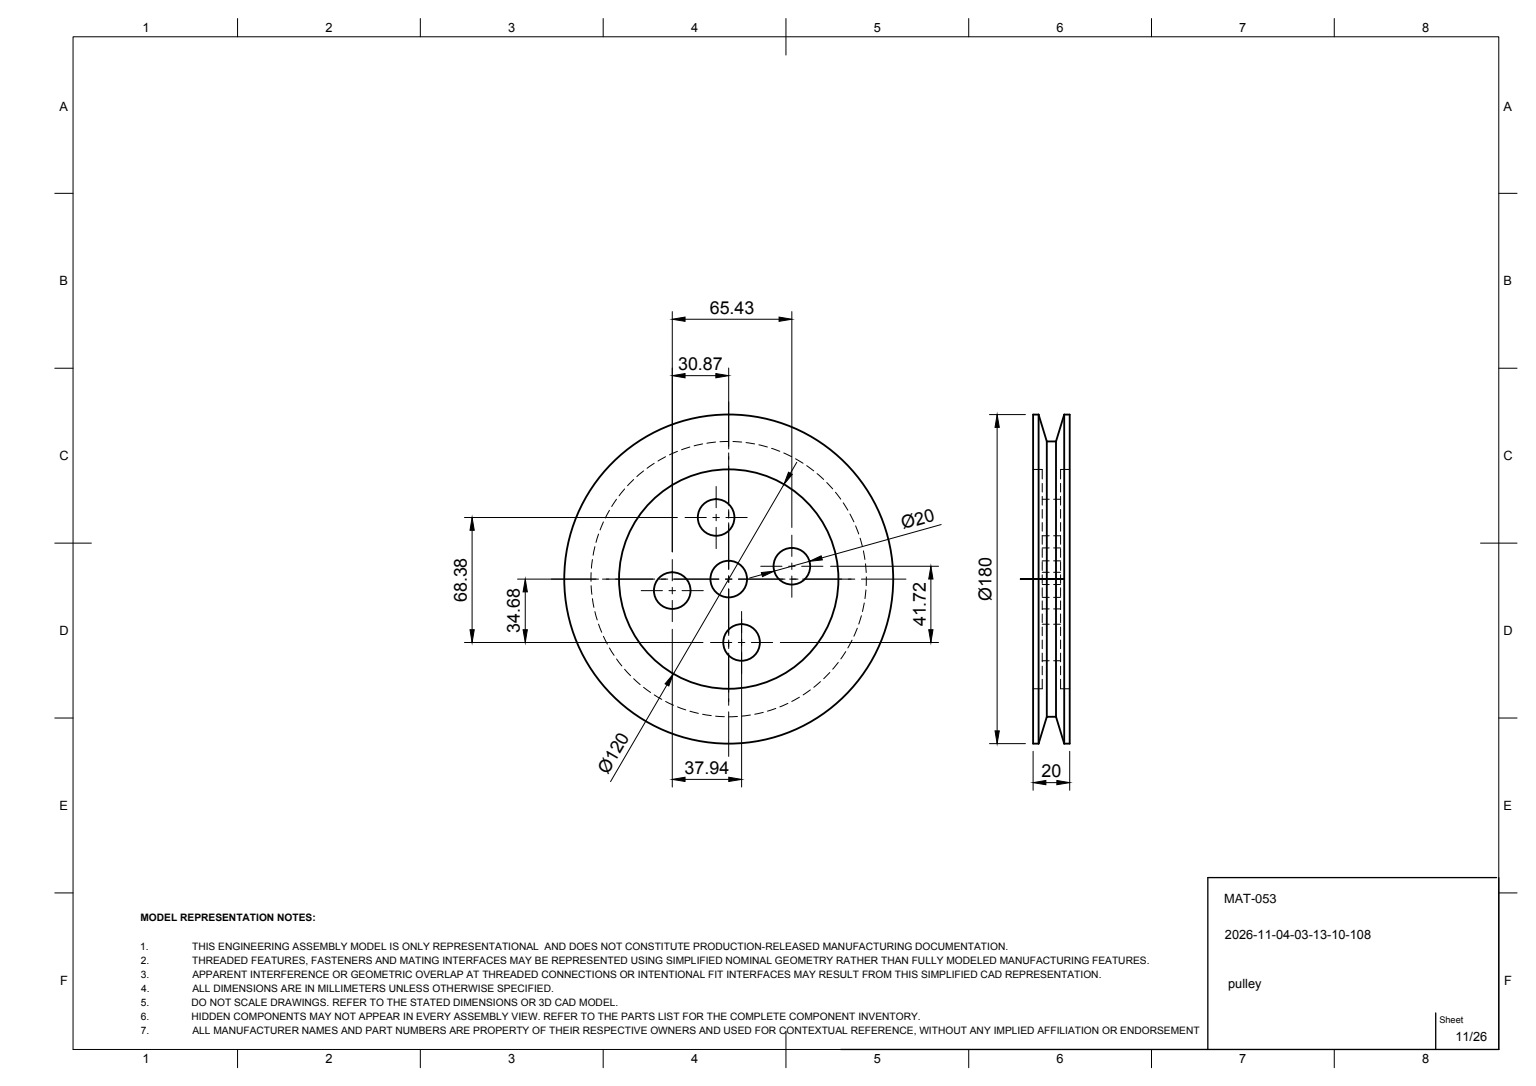
ISO-10303-21;
HEADER;
FILE_DESCRIPTION (('STEP AP214'),
    '1' );
FILE_NAME ('pulley.step',
    '2026-10-10T03:43:58',
    ( '' ),
    ( '' ),
    'SwSTEP 2.0',
    'SolidWorks 2026',
    '' );
FILE_SCHEMA (( 'AUTOMOTIVE_DESIGN' ));
ENDSEC;

DATA;
#61=CYLINDRICAL_SURFACE ( 'NONE', #28597, 10.00000000000000000 ) ;
#98=ORIENTED_EDGE ( 'NONE', *, *, #55652, .T. ) ;
#151=ADVANCED_FACE ( 'NONE', ( #63279 ), #44007, .T. ) ;
#319=CIRCLE ( 'NONE', #56472, 10.00000000000000178 ) ;
#365=AXIS2_PLACEMENT_3D ( 'NONE', #2334, #1994, #61414 ) ;
#474=DIRECTION ( 'NONE',  ( 0.000000000000000000, 0.000000000000000000, 1.000000000000000000 ) ) ;
#651=DIRECTION ( 'NONE',  ( -1.000000000000000000, 0.000000000000000000, 0.000000000000000000 ) ) ;
#941=EDGE_CURVE ( 'NONE', #52293, #21319, #16043, .T. ) ;
#1200=ORIENTED_EDGE ( 'NONE', *, *, #38790, .T. ) ;
#1261=DIRECTION ( 'NONE',  ( 0.000000000000000000, 0.000000000000000000, 1.000000000000000000 ) ) ;
#1262=EDGE_CURVE ( 'NONE', #23524, #39998, #319, .T. ) ;
#1394=( NAMED_UNIT ( * ) SI_UNIT ( $, .STERADIAN. ) SOLID_ANGLE_UNIT ( ) );
#1416=CARTESIAN_POINT ( 'NONE',  ( 0.000000000000000000, 35.26862320190615208, -9.999999999999998224 ) ) ;
#1462=CARTESIAN_POINT ( 'NONE',  ( 89.99999999999998579, 0.000000000000000000, 7.000000000000000000 ) ) ;
#1503=EDGE_LOOP ( 'NONE', ( #64737, #47138, #56812, #9323 ) ) ;
#1529=LINE ( 'NONE', #55690, #24184 ) ;
#1565=MECHANICAL_DESIGN_GEOMETRIC_PRESENTATION_REPRESENTATION('',(#34171),#59945);
#1694=EDGE_CURVE ( 'NONE', #53100, #28536, #21713, .T. ) ;
#1730=AXIS2_PLACEMENT_3D ( 'NONE', #16357, #31849, #58564 ) ;
#1752=FILL_AREA_STYLE ('',( #65780 ) ) ;
#1861=CARTESIAN_POINT ( 'NONE',  ( 0.000000000000000000, 0.000000000000000000, 10.00000000000000000 ) ) ;
#1994=DIRECTION ( 'NONE',  ( -0.000000000000000000, -0.000000000000000000, 1.000000000000000000 ) ) ;
#2049=DIRECTION ( 'NONE',  ( 1.000000000000000000, 0.000000000000000000, 0.000000000000000000 ) ) ;
#2163=EDGE_CURVE ( 'NONE', #30662, #53211, #9601, .T. ) ;
#2167=DIRECTION ( 'NONE',  ( 0.000000000000000000, 0.000000000000000000, 1.000000000000000000 ) ) ;
#2236=EDGE_CURVE ( 'NONE', #53211, #61781, #59915, .T. ) ;
#2298=AXIS2_PLACEMENT_3D ( 'NONE', #8382, #19975, #61496 ) ;
#2334=CARTESIAN_POINT ( 'NONE',  ( 0.000000000000000000, 0.000000000000000000, 2.500000000000030198 ) ) ;
#2371=EDGE_LOOP ( 'NONE', ( #59908, #20323, #39063, #20263 ) ) ;
#2403=VERTEX_POINT ( 'NONE', #29243 ) ;
#2428=CARTESIAN_POINT ( 'NONE',  ( -60.00000000000000000, 0.000000000000000000, -10.00000000000000000 ) ) ;
#2431=EDGE_LOOP ( 'NONE', ( #44600, #48576 ) ) ;
#2555=DIRECTION ( 'NONE',  ( 1.000000000000000000, 0.000000000000000000, 0.000000000000000000 ) ) ;
#2581=ORIENTED_EDGE ( 'NONE', *, *, #47265, .T. ) ;
#2644=ORIENTED_EDGE ( 'NONE', *, *, #1262, .F. ) ;
#2646=CIRCLE ( 'NONE', #56567, 60.00000000000000000 ) ;
#2656=DIRECTION ( 'NONE',  ( 0.000000000000000000, 0.000000000000000000, 1.000000000000000000 ) ) ;
#2718=DIRECTION ( 'NONE',  ( 1.000000000000000000, 0.000000000000000000, 0.000000000000000000 ) ) ;
#2740=AXIS2_PLACEMENT_3D ( 'NONE', #51849, #29706, #19145 ) ;
#2780=EDGE_CURVE ( 'NONE', #47684, #28536, #39364, .T. ) ;
#2790=ORIENTED_EDGE ( 'NONE', *, *, #64406, .T. ) ;
#2793=AXIS2_PLACEMENT_3D ( 'NONE', #21535, #48592, #64454 ) ;
#2893=VERTEX_POINT ( 'NONE', #68763 ) ;
#3121=EDGE_CURVE ( 'NONE', #10742, #65175, #4948, .T. ) ;
#3254=ADVANCED_FACE ( 'NONE', ( #52841, #58140 ), #58814, .F. ) ;
#3361=CARTESIAN_POINT ( 'NONE',  ( -10.00000000000000178, -31.50328976398030534, -5.000000000000000000 ) ) ;
#3370=ORIENTED_EDGE ( 'NONE', *, *, #2236, .F. ) ;
#3553=ORIENTED_EDGE ( 'NONE', *, *, #22471, .F. ) ;
#3589=VECTOR ( 'NONE', #31637, 1000.000000000000000 ) ;
#3744=EDGE_LOOP ( 'NONE', ( #59233, #13673, #7017, #48460 ) ) ;
#3816=CARTESIAN_POINT ( 'NONE',  ( 0.000000000000000000, 0.000000000000000000, -5.000000000000000000 ) ) ;
#3870=ORIENTED_EDGE ( 'NONE', *, *, #47160, .T. ) ;
#4067=DIRECTION ( 'NONE',  ( -0.000000000000000000, -0.000000000000000000, 1.000000000000000000 ) ) ;
#4088=SHAPE_DEFINITION_REPRESENTATION ( #20886, #7414 ) ;
#4166=FACE_BOUND ( 'NONE', #26669, .T. ) ;
#4396=CARTESIAN_POINT ( 'NONE',  ( 0.000000000000000000, 35.26862320190615208, -5.000000000000000000 ) ) ;
#4448=DIRECTION ( 'NONE',  ( -0.000000000000000000, -0.000000000000000000, -1.000000000000000000 ) ) ;
#4451=ORIENTED_EDGE ( 'NONE', *, *, #11819, .F. ) ;
#4637=AXIS2_PLACEMENT_3D ( 'NONE', #21081, #17074, #49079 ) ;
#4684=AXIS2_PLACEMENT_3D ( 'NONE', #58250, #22002, #20968 ) ;
#4704=EDGE_CURVE ( 'NONE', #10742, #21319, #42324, .T. ) ;
#4769=EDGE_LOOP ( 'NONE', ( #6850, #46312, #5479, #66133 ) ) ;
#4782=CARTESIAN_POINT ( 'NONE',  ( 0.000000000000000000, 0.000000000000000000, 2.500000000000030198 ) ) ;
#4843=FACE_OUTER_BOUND ( 'NONE', #65401, .T. ) ;
#4888=VECTOR ( 'NONE', #64816, 1000.000000000000000 ) ;
#4897=EDGE_CURVE ( 'NONE', #66948, #13402, #48184, .T. ) ;
#4914=EDGE_CURVE ( 'NONE', #2403, #18591, #2646, .T. ) ;
#4948=CIRCLE ( 'NONE', #10407, 10.00000000000000178 ) ;
#5011=CARTESIAN_POINT ( 'NONE',  ( 0.000000000000000000, 0.000000000000000000, -10.00000000000000000 ) ) ;
#5069=ORIENTED_EDGE ( 'NONE', *, *, #52323, .T. ) ;
#5081=CARTESIAN_POINT ( 'NONE',  ( 35.39413431650373099, 0.000000000000000000, -9.999999999999998224 ) ) ;
#5354=DIRECTION ( 'NONE',  ( 1.000000000000000000, 0.000000000000000000, 0.000000000000000000 ) ) ;
#5479=ORIENTED_EDGE ( 'NONE', *, *, #19013, .F. ) ;
#5630=CARTESIAN_POINT ( 'NONE',  ( 89.99999999999998579, 0.000000000000000000, 7.000000000000000000 ) ) ;
#5730=AXIS2_PLACEMENT_3D ( 'NONE', #1861, #22599, #60236 ) ;
#5982=VECTOR ( 'NONE', #10217, 999.9999999999998863 ) ;
#6135=AXIS2_PLACEMENT_3D ( 'NONE', #10751, #4448, #36807 ) ;
#6243=ORIENTED_EDGE ( 'NONE', *, *, #19527, .T. ) ;
#6270=ORIENTED_EDGE ( 'NONE', *, *, #4897, .F. ) ;
#6271=EDGE_LOOP ( 'NONE', ( #58574, #4451 ) ) ;
#6334=DIRECTION ( 'NONE',  ( 0.000000000000000000, 0.000000000000000000, 1.000000000000000000 ) ) ;
#6410=ADVANCED_FACE ( 'NONE', ( #50308 ), #22872, .F. ) ;
#6426=ORIENTED_EDGE ( 'NONE', *, *, #48732, .T. ) ;
#6486=AXIS2_PLACEMENT_3D ( 'NONE', #11579, #27769, #7377 ) ;
#6559=LINE ( 'NONE', #26464, #41857 ) ;
#6569=DIRECTION ( 'NONE',  ( 1.000000000000000000, 0.000000000000000000, 0.000000000000000000 ) ) ;
#6575=CYLINDRICAL_SURFACE ( 'NONE', #36283, 10.00000000000000178 ) ;
#6794=VERTEX_POINT ( 'NONE', #69156 ) ;
#6834=CARTESIAN_POINT ( 'NONE',  ( 0.000000000000000000, -31.50328976398030534, -9.999999999999998224 ) ) ;
#6850=ORIENTED_EDGE ( 'NONE', *, *, #7053, .T. ) ;
#6887=CARTESIAN_POINT ( 'NONE',  ( 89.99999999999998579, 0.000000000000000000, -7.000000000000000000 ) ) ;
#6996=LINE ( 'NONE', #34089, #60070 ) ;
#7017=ORIENTED_EDGE ( 'NONE', *, *, #941, .T. ) ;
#7039=DIRECTION ( 'NONE',  ( -0.000000000000000000, -0.000000000000000000, 1.000000000000000000 ) ) ;
#7047=EDGE_CURVE ( 'NONE', #45363, #9869, #62339, .T. ) ;
#7053=EDGE_CURVE ( 'NONE', #68618, #30662, #37622, .T. ) ;
#7236=EDGE_CURVE ( 'NONE', #21145, #17425, #50034, .T. ) ;
#7241=DIRECTION ( 'NONE',  ( 1.000000000000000000, 0.000000000000000000, 0.000000000000000000 ) ) ;
#7247=ORIENTED_EDGE ( 'NONE', *, *, #41042, .T. ) ;
#7317=AXIS2_PLACEMENT_3D ( 'NONE', #58860, #10002, #69423 ) ;
#7333=ORIENTED_EDGE ( 'NONE', *, *, #46538, .F. ) ;
#7377=DIRECTION ( 'NONE',  ( 1.000000000000000000, 0.000000000000000000, 0.000000000000000000 ) ) ;
#7414=SHAPE_REPRESENTATION ( 'pulley', ( #66832 ), #23071 ) ;
#7453=DIRECTION ( 'NONE',  ( 1.000000000000000000, 0.000000000000000000, 0.000000000000000000 ) ) ;
#7463=EDGE_CURVE ( 'NONE', #12451, #43150, #55952, .T. ) ;
#7697=AXIS2_PLACEMENT_3D ( 'NONE', #38245, #42146, #53030 ) ;
#7758=DIRECTION ( 'NONE',  ( 1.000000000000000000, 0.000000000000000000, 0.000000000000000000 ) ) ;
#7775=CARTESIAN_POINT ( 'NONE',  ( -44.39004539972346208, 1.224646799147353059E-15, 5.000000000000000000 ) ) ;
#7976=EDGE_LOOP ( 'NONE', ( #6270, #47375, #12404, #6426 ) ) ;
#8319=DIRECTION ( 'NONE',  ( 1.000000000000000000, 0.000000000000000000, 0.000000000000000000 ) ) ;
#8359=ADVANCED_FACE ( 'NONE', ( #59050, #26025, #42538, #37948, #37249, #31988 ), #26369, .T. ) ;
#8382=CARTESIAN_POINT ( 'NONE',  ( 0.000000000000000000, 0.000000000000000000, -50.00000000000000711 ) ) ;
#8432=ADVANCED_FACE ( 'NONE', ( #11546 ), #33731, .F. ) ;
#8454=CARTESIAN_POINT ( 'NONE',  ( -34.39004539972345498, 0.000000000000000000, -9.999999999999998224 ) ) ;
#8513=CARTESIAN_POINT ( 'NONE',  ( 89.99999999999998579, 0.000000000000000000, 10.00000000000000000 ) ) ;
#8624=EDGE_CURVE ( 'NONE', #11248, #10057, #61672, .T. ) ;
#8655=ORIENTED_EDGE ( 'NONE', *, *, #46300, .T. ) ;
#8682=ORIENTED_EDGE ( 'NONE', *, *, #41042, .F. ) ;
#8921=AXIS2_PLACEMENT_3D ( 'NONE', #60437, #34420, #651 ) ;
#8935=ORIENTED_EDGE ( 'NONE', *, *, #27892, .T. ) ;
#9037=CARTESIAN_POINT ( 'NONE',  ( 0.000000000000000000, -31.50328976398030534, 5.000000000000000000 ) ) ;
#9296=DIRECTION ( 'NONE',  ( -0.000000000000000000, -0.000000000000000000, 1.000000000000000000 ) ) ;
#9299=CARTESIAN_POINT ( 'NONE',  ( -60.00000000000000000, 7.347880794884118356E-15, 5.000000000000000000 ) ) ;
#9323=ORIENTED_EDGE ( 'NONE', *, *, #67194, .F. ) ;
#9353=ADVANCED_FACE ( 'NONE', ( #51360 ), #35525, .T. ) ;
#9510=DIRECTION ( 'NONE',  ( 0.000000000000000000, 0.000000000000000000, 1.000000000000000000 ) ) ;
#9547=VERTEX_POINT ( 'NONE', #49508 ) ;
#9601=LINE ( 'NONE', #31064, #27333 ) ;
#9685=ORIENTED_EDGE ( 'NONE', *, *, #17023, .T. ) ;
#9689=DIRECTION ( 'NONE',  ( 0.000000000000000000, 0.000000000000000000, 1.000000000000000000 ) ) ;
#9869=VERTEX_POINT ( 'NONE', #16396 ) ;
#10002=DIRECTION ( 'NONE',  ( -0.000000000000000000, -0.000000000000000000, 1.000000000000000000 ) ) ;
#10051=VECTOR ( 'NONE', #40595, 1000.000000000000000 ) ;
#10057=VERTEX_POINT ( 'NONE', #36395 ) ;
#10178=CARTESIAN_POINT ( 'NONE',  ( 0.000000000000000000, 0.000000000000000000, 5.000000000000000000 ) ) ;
#10217=DIRECTION ( 'NONE',  ( 0.9561276726666709802, 1.170918693907447064E-16, -0.2929502919626733037 ) ) ;
#10257=AXIS2_PLACEMENT_3D ( 'NONE', #8454, #17612, #17965 ) ;
#10407=AXIS2_PLACEMENT_3D ( 'NONE', #35304, #56760, #35656 ) ;
#10513=DIRECTION ( 'NONE',  ( 1.000000000000000000, 0.000000000000000000, 0.000000000000000000 ) ) ;
#10545=ORIENTED_EDGE ( 'NONE', *, *, #941, .F. ) ;
#10712=LINE ( 'NONE', #53950, #37950 ) ;
#10742=VERTEX_POINT ( 'NONE', #35449 ) ;
#10751=CARTESIAN_POINT ( 'NONE',  ( 0.000000000000000000, 0.000000000000000000, -5.000000000000000000 ) ) ;
#10829=EDGE_LOOP ( 'NONE', ( #67970, #52613, #98, #33206 ) ) ;
#10892=ORIENTED_EDGE ( 'NONE', *, *, #33419, .T. ) ;
#11059=CARTESIAN_POINT ( 'NONE',  ( -10.00000000000000000, 1.224646799147353256E-15, -50.00000000000000711 ) ) ;
#11248=VERTEX_POINT ( 'NONE', #3361 ) ;
#11305=CARTESIAN_POINT ( 'NONE',  ( 0.000000000000000000, 0.000000000000000000, -50.00000000000000711 ) ) ;
#11354=DIRECTION ( 'NONE',  ( 1.000000000000000000, 0.000000000000000000, 0.000000000000000000 ) ) ;
#11546=FACE_OUTER_BOUND ( 'NONE', #63868, .T. ) ;
#11579=CARTESIAN_POINT ( 'NONE',  ( 0.000000000000000000, 0.000000000000000000, -10.00000000000000000 ) ) ;
#11681=ORIENTED_EDGE ( 'NONE', *, *, #47864, .F. ) ;
#11757=DIRECTION ( 'NONE',  ( 1.000000000000000000, 0.000000000000000000, 0.000000000000000000 ) ) ;
#11819=EDGE_CURVE ( 'NONE', #30259, #53637, #18799, .T. ) ;
#11950=DIRECTION ( 'NONE',  ( -0.000000000000000000, -0.000000000000000000, 1.000000000000000000 ) ) ;
#12100=EDGE_CURVE ( 'NONE', #2893, #44947, #27719, .T. ) ;
#12102=DIRECTION ( 'NONE',  ( 1.000000000000000000, 0.000000000000000000, 0.000000000000000000 ) ) ;
#12106=ORIENTED_EDGE ( 'NONE', *, *, #38790, .F. ) ;
#12276=CARTESIAN_POINT ( 'NONE',  ( 0.000000000000000000, 0.000000000000000000, -5.000000000000000000 ) ) ;
#12300=SURFACE_STYLE_FILL_AREA ( #1752 ) ;
#12372=FACE_OUTER_BOUND ( 'NONE', #13779, .T. ) ;
#12404=ORIENTED_EDGE ( 'NONE', *, *, #67194, .T. ) ;
#12410=ORIENTED_EDGE ( 'NONE', *, *, #55652, .F. ) ;
#12451=VERTEX_POINT ( 'NONE', #50090 ) ;
#12519=CARTESIAN_POINT ( 'NONE',  ( -34.39004539972345498, 0.000000000000000000, 5.000000000000000000 ) ) ;
#12551=FACE_OUTER_BOUND ( 'NONE', #3744, .T. ) ;
#12617=EDGE_LOOP ( 'NONE', ( #21075, #40042 ) ) ;
#12653=PRESENTATION_STYLE_ASSIGNMENT (( #29179 ) ) ;
#12808=EDGE_LOOP ( 'NONE', ( #2644, #35837 ) ) ;
#12934=CARTESIAN_POINT ( 'NONE',  ( 0.000000000000000000, -31.50328976398030534, -9.999999999999998224 ) ) ;
#13038=CIRCLE ( 'NONE', #25394, 10.00000000000000178 ) ;
#13049=FACE_OUTER_BOUND ( 'NONE', #2371, .T. ) ;
#13176=CIRCLE ( 'NONE', #36765, 60.00000000000000000 ) ;
#13196=ORIENTED_EDGE ( 'NONE', *, *, #60306, .F. ) ;
#13220=DIRECTION ( 'NONE',  ( 1.000000000000000000, 0.000000000000000000, 0.000000000000000000 ) ) ;
#13374=CARTESIAN_POINT ( 'NONE',  ( -89.99999999999998579, 1.102182119232617596E-14, 7.000000000000000000 ) ) ;
#13402=VERTEX_POINT ( 'NONE', #6887 ) ;
#13464=VECTOR ( 'NONE', #31449, 1000.000000000000000 ) ;
#13673=ORIENTED_EDGE ( 'NONE', *, *, #49690, .T. ) ;
#13697=LINE ( 'NONE', #49932, #55890 ) ;
#13724=CARTESIAN_POINT ( 'NONE',  ( 10.00000000000000178, -31.50328976398030534, -9.999999999999998224 ) ) ;
#13779=EDGE_LOOP ( 'NONE', ( #39660, #49194, #20199, #56429 ) ) ;
#13918=EDGE_LOOP ( 'NONE', ( #29003, #10892, #68043, #19610 ) ) ;
#13923=CARTESIAN_POINT ( 'NONE',  ( -75.31295361348102801, 9.223176757708264319E-15, 2.500000000000030198 ) ) ;
#14038=VECTOR ( 'NONE', #9296, 1000.000000000000000 ) ;
#14075=EDGE_CURVE ( 'NONE', #50425, #20755, #16062, .T. ) ;
#14430=AXIS2_PLACEMENT_3D ( 'NONE', #16488, #59392, #10513 ) ;
#14504=ADVANCED_FACE ( 'NONE', ( #20920 ), #64168, .F. ) ;
#14523=CIRCLE ( 'NONE', #25733, 10.00000000000000178 ) ;
#14612=DIRECTION ( 'NONE',  ( 1.000000000000000000, 0.000000000000000000, 0.000000000000000000 ) ) ;
#14735=DIRECTION ( 'NONE',  ( -0.000000000000000000, -0.000000000000000000, 1.000000000000000000 ) ) ;
#14817=AXIS2_PLACEMENT_3D ( 'NONE', #9037, #51934, #2718 ) ;
#14996=CYLINDRICAL_SURFACE ( 'NONE', #6135, 60.00000000000000000 ) ;
#15212=LINE ( 'NONE', #52828, #51280 ) ;
#15564=DIRECTION ( 'NONE',  ( -0.000000000000000000, -0.000000000000000000, 1.000000000000000000 ) ) ;
#15578=PRODUCT_DEFINITION_CONTEXT ( 'detailed design', #55716, 'design' ) ;
#15691=FACE_OUTER_BOUND ( 'NONE', #46295, .T. ) ;
#15971=DIRECTION ( 'NONE',  ( -1.000000000000000000, 0.000000000000000000, 0.000000000000000000 ) ) ;
#16043=CIRCLE ( 'NONE', #57638, 10.00000000000000178 ) ;
#16062=LINE ( 'NONE', #58619, #49377 ) ;
#16244=EDGE_CURVE ( 'NONE', #6794, #27439, #31571, .T. ) ;
#16357=CARTESIAN_POINT ( 'NONE',  ( 0.000000000000000000, 0.000000000000000000, -10.00000000000000000 ) ) ;
#16396=CARTESIAN_POINT ( 'NONE',  ( -89.99999999999998579, 1.102182119232617596E-14, -10.00000000000000000 ) ) ;
#16488=CARTESIAN_POINT ( 'NONE',  ( 0.000000000000000000, 0.000000000000000000, -10.00000000000000000 ) ) ;
#16557=AXIS2_PLACEMENT_3D ( 'NONE', #18172, #45239, #6569 ) ;
#16580=ORIENTED_EDGE ( 'NONE', *, *, #2780, .F. ) ;
#16619=AXIS2_PLACEMENT_3D ( 'NONE', #39594, #2656, #40976 ) ;
#16620=ORIENTED_EDGE ( 'NONE', *, *, #51700, .F. ) ;
#16686=EDGE_CURVE ( 'NONE', #66948, #47684, #54082, .T. ) ;
#16809=LINE ( 'NONE', #49156, #47554 ) ;
#17023=EDGE_CURVE ( 'NONE', #44947, #9547, #6996, .T. ) ;
#17037=CYLINDRICAL_SURFACE ( 'NONE', #1730, 89.99999999999998579 ) ;
#17074=DIRECTION ( 'NONE',  ( 0.000000000000000000, 0.000000000000000000, 1.000000000000000000 ) ) ;
#17125=AXIS2_PLACEMENT_3D ( 'NONE', #54806, #50934, #23164 ) ;
#17213=CARTESIAN_POINT ( 'NONE',  ( 60.00000000000000000, 0.000000000000000000, 5.000000000000000000 ) ) ;
#17290=CARTESIAN_POINT ( 'NONE',  ( 35.39413431650373099, 0.000000000000000000, -5.000000000000000000 ) ) ;
#17382=FACE_OUTER_BOUND ( 'NONE', #10829, .T. ) ;
#17425=VERTEX_POINT ( 'NONE', #61678 ) ;
#17612=DIRECTION ( 'NONE',  ( -0.000000000000000000, -0.000000000000000000, 1.000000000000000000 ) ) ;
#17645=DIRECTION ( 'NONE',  ( 1.000000000000000000, 0.000000000000000000, 0.000000000000000000 ) ) ;
#17965=DIRECTION ( 'NONE',  ( 1.000000000000000000, 0.000000000000000000, 0.000000000000000000 ) ) ;
#18029=DIRECTION ( 'NONE',  ( 0.000000000000000000, 0.000000000000000000, 1.000000000000000000 ) ) ;
#18172=CARTESIAN_POINT ( 'NONE',  ( 0.000000000000000000, 0.000000000000000000, -10.00000000000000000 ) ) ;
#18202=EDGE_CURVE ( 'NONE', #17425, #2403, #29517, .T. ) ;
#18545=ORIENTED_EDGE ( 'NONE', *, *, #34312, .F. ) ;
#18587=CONICAL_SURFACE ( 'NONE', #42136, 75.31295361348104223, 1.273485274044411586 ) ;
#18591=VERTEX_POINT ( 'NONE', #67778 ) ;
#18605=ORIENTED_EDGE ( 'NONE', *, *, #3121, .F. ) ;
#18616=VECTOR ( 'NONE', #52054, 1000.000000000000000 ) ;
#18687=CARTESIAN_POINT ( 'NONE',  ( 0.000000000000000000, 0.000000000000000000, 10.00000000000000000 ) ) ;
#18709=VECTOR ( 'NONE', #66024, 1000.000000000000000 ) ;
#18799=CIRCLE ( 'NONE', #42345, 10.00000000000000178 ) ;
#18919=CARTESIAN_POINT ( 'NONE',  ( 10.00000000000000178, -31.50328976398030534, 5.000000000000000000 ) ) ;
#18926=CARTESIAN_POINT ( 'NONE',  ( -60.00000000000000000, 7.347880794884118356E-15, 5.000000000000000000 ) ) ;
#18993=CARTESIAN_POINT ( 'NONE',  ( 0.000000000000000000, 0.000000000000000000, 10.00000000000000000 ) ) ;
#19013=EDGE_CURVE ( 'NONE', #61781, #53211, #19248, .T. ) ;
#19145=DIRECTION ( 'NONE',  ( 1.000000000000000000, 0.000000000000000000, 0.000000000000000000 ) ) ;
#19248=CIRCLE ( 'NONE', #5730, 89.99999999999998579 ) ;
#19463=EDGE_CURVE ( 'NONE', #20755, #30529, #57469, .T. ) ;
#19525=DIRECTION ( 'NONE',  ( 0.000000000000000000, 0.000000000000000000, 1.000000000000000000 ) ) ;
#19527=EDGE_CURVE ( 'NONE', #47684, #66948, #67617, .T. ) ;
#19586=EDGE_CURVE ( 'NONE', #28536, #53100, #60827, .T. ) ;
#19610=ORIENTED_EDGE ( 'NONE', *, *, #18202, .F. ) ;
#19678=DIRECTION ( 'NONE',  ( 0.000000000000000000, 0.000000000000000000, 1.000000000000000000 ) ) ;
#19778=DIRECTION ( 'NONE',  ( 0.000000000000000000, 0.000000000000000000, 1.000000000000000000 ) ) ;
#19800=CIRCLE ( 'NONE', #46751, 60.00000000000000000 ) ;
#19975=DIRECTION ( 'NONE',  ( -0.000000000000000000, -0.000000000000000000, 1.000000000000000000 ) ) ;
#20066=CARTESIAN_POINT ( 'NONE',  ( 35.39413431650373099, 0.000000000000000000, 5.000000000000000000 ) ) ;
#20199=ORIENTED_EDGE ( 'NONE', *, *, #18202, .T. ) ;
#20233=DIRECTION ( 'NONE',  ( -1.000000000000000000, 0.000000000000000000, 0.000000000000000000 ) ) ;
#20263=ORIENTED_EDGE ( 'NONE', *, *, #40347, .T. ) ;
#20321=AXIS2_PLACEMENT_3D ( 'NONE', #4396, #36753, #36062 ) ;
#20323=ORIENTED_EDGE ( 'NONE', *, *, #34312, .T. ) ;
#20358=EDGE_LOOP ( 'NONE', ( #40227, #3870 ) ) ;
#20755=VERTEX_POINT ( 'NONE', #40805 ) ;
#20828=ORIENTED_EDGE ( 'NONE', *, *, #47858, .T. ) ;
#20886=PRODUCT_DEFINITION_SHAPE ( 'NONE', 'NONE',  #57716 ) ;
#20920=FACE_OUTER_BOUND ( 'NONE', #24665, .T. ) ;
#20955=EDGE_CURVE ( 'NONE', #39170, #22725, #44086, .T. ) ;
#20968=DIRECTION ( 'NONE',  ( 1.000000000000000000, 0.000000000000000000, 0.000000000000000000 ) ) ;
#21075=ORIENTED_EDGE ( 'NONE', *, *, #7047, .F. ) ;
#21081=CARTESIAN_POINT ( 'NONE',  ( 0.000000000000000000, 0.000000000000000000, 5.000000000000000000 ) ) ;
#21136=ORIENTED_EDGE ( 'NONE', *, *, #19463, .F. ) ;
#21145=VERTEX_POINT ( 'NONE', #18926 ) ;
#21198=DIRECTION ( 'NONE',  ( 1.000000000000000000, 0.000000000000000000, -0.000000000000000000 ) ) ;
#21199=CIRCLE ( 'NONE', #60511, 10.00000000000000000 ) ;
#21283=DIRECTION ( 'NONE',  ( -1.000000000000000000, 0.000000000000000000, 0.000000000000000000 ) ) ;
#21319=VERTEX_POINT ( 'NONE', #63564 ) ;
#21446=AXIS2_PLACEMENT_3D ( 'NONE', #60287, #64868, #12102 ) ;
#21521=DIRECTION ( 'NONE',  ( 0.000000000000000000, 0.000000000000000000, 1.000000000000000000 ) ) ;
#21535=CARTESIAN_POINT ( 'NONE',  ( 0.000000000000000000, 0.000000000000000000, 7.000000000000000000 ) ) ;
#21581=CARTESIAN_POINT ( 'NONE',  ( 60.00000000000000000, 7.347880794884118356E-15, -5.000000000000000000 ) ) ;
#21713=CIRCLE ( 'NONE', #365, 75.31295361348102801 ) ;
#21837=ADVANCED_FACE ( 'NONE', ( #24401 ), #47815, .F. ) ;
#21846=CYLINDRICAL_SURFACE ( 'NONE', #31458, 89.99999999999998579 ) ;
#21868=EDGE_LOOP ( 'NONE', ( #34452, #7247, #37847, #29975 ) ) ;
#22002=DIRECTION ( 'NONE',  ( -0.000000000000000000, -0.000000000000000000, 1.000000000000000000 ) ) ;
#22054=DIRECTION ( 'NONE',  ( 1.000000000000000000, 0.000000000000000000, 0.000000000000000000 ) ) ;
#22124=CARTESIAN_POINT ( 'NONE',  ( 0.000000000000000000, 0.000000000000000000, -5.000000000000000000 ) ) ;
#22395=VECTOR ( 'NONE', #29536, 1000.000000000000227 ) ;
#22413=CIRCLE ( 'NONE', #8921, 10.00000000000000178 ) ;
#22471=EDGE_CURVE ( 'NONE', #30662, #68618, #37511, .T. ) ;
#22485=ORIENTED_EDGE ( 'NONE', *, *, #41632, .F. ) ;
#22599=DIRECTION ( 'NONE',  ( 0.000000000000000000, 0.000000000000000000, 1.000000000000000000 ) ) ;
#22637=FACE_OUTER_BOUND ( 'NONE', #1503, .T. ) ;
#22725=VERTEX_POINT ( 'NONE', #58137 ) ;
#22787=EDGE_LOOP ( 'NONE', ( #28842, #20828, #57321, #33604 ) ) ;
#22810=DIRECTION ( 'NONE',  ( -1.000000000000000000, 0.000000000000000000, 0.000000000000000000 ) ) ;
#22872=CYLINDRICAL_SURFACE ( 'NONE', #58908, 10.00000000000000178 ) ;
#22964=AXIS2_PLACEMENT_3D ( 'NONE', #60027, #66039, #32956 ) ;
#23071=( GEOMETRIC_REPRESENTATION_CONTEXT ( 3 ) GLOBAL_UNCERTAINTY_ASSIGNED_CONTEXT ( ( #68356 ) ) GLOBAL_UNIT_ASSIGNED_CONTEXT ( ( #36345, #41619, #46543 ) ) REPRESENTATION_CONTEXT ( 'NONE', 'WORKASPACE' ) );
#23164=DIRECTION ( 'NONE',  ( -1.000000000000000000, 0.000000000000000000, 0.000000000000000000 ) ) ;
#23251=CYLINDRICAL_SURFACE ( 'NONE', #10257, 10.00000000000000178 ) ;
#23524=VERTEX_POINT ( 'NONE', #38498 ) ;
#23619=DIRECTION ( 'NONE',  ( 1.000000000000000000, 0.000000000000000000, 0.000000000000000000 ) ) ;
#23675=ORIENTED_EDGE ( 'NONE', *, *, #64054, .F. ) ;
#23979=DIRECTION ( 'NONE',  ( 0.000000000000000000, 0.000000000000000000, -1.000000000000000000 ) ) ;
#24000=LINE ( 'NONE', #60933, #30651 ) ;
#24087=ORIENTED_EDGE ( 'NONE', *, *, #64141, .T. ) ;
#24106=LINE ( 'NONE', #57489, #14038 ) ;
#24184=VECTOR ( 'NONE', #55334, 1000.000000000000000 ) ;
#24314=ADVANCED_FACE ( 'NONE', ( #58147 ), #44339, .T. ) ;
#24401=FACE_OUTER_BOUND ( 'NONE', #39768, .T. ) ;
#24665=EDGE_LOOP ( 'NONE', ( #43122, #49749, #68545, #49224 ) ) ;
#24720=DIRECTION ( 'NONE',  ( 1.000000000000000000, 0.000000000000000000, 0.000000000000000000 ) ) ;
#24744=DIRECTION ( 'NONE',  ( -1.000000000000000000, 0.000000000000000000, 0.000000000000000000 ) ) ;
#24810=CARTESIAN_POINT ( 'NONE',  ( 0.000000000000000000, 0.000000000000000000, -7.000000000000000000 ) ) ;
#24873=CARTESIAN_POINT ( 'NONE',  ( -10.00000000000000000, 1.224646799147353256E-15, -4.999999999999997335 ) ) ;
#24889=ADVANCED_FACE ( 'NONE', ( #64197 ), #17037, .T. ) ;
#25312=ORIENTED_EDGE ( 'NONE', *, *, #16244, .T. ) ;
#25394=AXIS2_PLACEMENT_3D ( 'NONE', #26904, #42732, #21283 ) ;
#25533=DIRECTION ( 'NONE',  ( 1.000000000000000000, 0.000000000000000000, 0.000000000000000000 ) ) ;
#25733=AXIS2_PLACEMENT_3D ( 'NONE', #66482, #65782, #29181 ) ;
#25747=EDGE_CURVE ( 'NONE', #53100, #68618, #59439, .T. ) ;
#25871=CARTESIAN_POINT ( 'NONE',  ( 0.000000000000000000, 0.000000000000000000, 7.000000000000000000 ) ) ;
#25997=CIRCLE ( 'NONE', #4637, 10.00000000000000000 ) ;
#26025=FACE_BOUND ( 'NONE', #6271, .T. ) ;
#26047=AXIS2_PLACEMENT_3D ( 'NONE', #24810, #68075, #13220 ) ;
#26119=ORIENTED_EDGE ( 'NONE', *, *, #52323, .F. ) ;
#26369=PLANE ( 'NONE',  #35485 ) ;
#26464=CARTESIAN_POINT ( 'NONE',  ( 25.39413431650373099, 1.224646799147353256E-15, -9.999999999999998224 ) ) ;
#26476=CARTESIAN_POINT ( 'NONE',  ( 25.39413431650373099, 1.224646799147353059E-15, 5.000000000000000000 ) ) ;
#26496=CARTESIAN_POINT ( 'NONE',  ( -44.39004539972346208, 1.224646799147353059E-15, -5.000000000000000000 ) ) ;
#26547=DIRECTION ( 'NONE',  ( 1.000000000000000000, 0.000000000000000000, 0.000000000000000000 ) ) ;
#26653=ORIENTED_EDGE ( 'NONE', *, *, #2163, .F. ) ;
#26666=CIRCLE ( 'NONE', #16557, 60.00000000000000000 ) ;
#26669=EDGE_LOOP ( 'NONE', ( #22485, #26976 ) ) ;
#26729=EDGE_LOOP ( 'NONE', ( #26653, #60522, #8655, #3370 ) ) ;
#26855=EDGE_LOOP ( 'NONE', ( #39743, #43103, #60080, #60764 ) ) ;
#26904=CARTESIAN_POINT ( 'NONE',  ( 0.000000000000000000, -31.50328976398030534, -5.000000000000000000 ) ) ;
#26976=ORIENTED_EDGE ( 'NONE', *, *, #64141, .F. ) ;
#27069=CARTESIAN_POINT ( 'NONE',  ( -10.00000000000000000, 1.224646799147353256E-15, 5.000000000000000000 ) ) ;
#27333=VECTOR ( 'NONE', #21521, 1000.000000000000000 ) ;
#27439=VERTEX_POINT ( 'NONE', #57091 ) ;
#27547=ORIENTED_EDGE ( 'NONE', *, *, #66502, .T. ) ;
#27719=CIRCLE ( 'NONE', #53569, 60.00000000000000000 ) ;
#27769=DIRECTION ( 'NONE',  ( 0.000000000000000000, 0.000000000000000000, 1.000000000000000000 ) ) ;
#27826=DIRECTION ( 'NONE',  ( 1.000000000000000000, 0.000000000000000000, 0.000000000000000000 ) ) ;
#27887=ORIENTED_EDGE ( 'NONE', *, *, #51784, .F. ) ;
#27892=EDGE_CURVE ( 'NONE', #44947, #2893, #66917, .T. ) ;
#27936=ORIENTED_EDGE ( 'NONE', *, *, #63523, .T. ) ;
#27949=EDGE_CURVE ( 'NONE', #17425, #21145, #19800, .T. ) ;
#28018=CARTESIAN_POINT ( 'NONE',  ( -75.31295361348104223, 0.000000000000000000, -2.499999999999970246 ) ) ;
#28120=SURFACE_SIDE_STYLE ('',( #12300 ) ) ;
#28344=DIRECTION ( 'NONE',  ( 1.000000000000000000, 0.000000000000000000, 0.000000000000000000 ) ) ;
#28475=( NAMED_UNIT ( * ) PLANE_ANGLE_UNIT ( ) SI_UNIT ( $, .RADIAN. ) );
#28536=VERTEX_POINT ( 'NONE', #13923 ) ;
#28597=AXIS2_PLACEMENT_3D ( 'NONE', #11305, #38754, #17645 ) ;
#28623=EDGE_LOOP ( 'NONE', ( #33068, #12410 ) ) ;
#28842=ORIENTED_EDGE ( 'NONE', *, *, #41632, .T. ) ;
#28936=EDGE_LOOP ( 'NONE', ( #18605, #18545 ) ) ;
#29003=ORIENTED_EDGE ( 'NONE', *, *, #7236, .F. ) ;
#29179=SURFACE_STYLE_USAGE ( .BOTH. , #28120 ) ;
#29181=DIRECTION ( 'NONE',  ( -1.000000000000000000, 0.000000000000000000, 0.000000000000000000 ) ) ;
#29235=ADVANCED_FACE ( 'NONE', ( #42134, #68527, #52348, #52680, #4166, #4843 ), #37542, .T. ) ;
#29243=CARTESIAN_POINT ( 'NONE',  ( 60.00000000000000000, 0.000000000000000000, 10.00000000000000000 ) ) ;
#29517=LINE ( 'NONE', #17213, #59598 ) ;
#29536=DIRECTION ( 'NONE',  ( -0.9561276726666719794, 1.170918693907448050E-16, 0.2929502919626694180 ) ) ;
#29537=FACE_OUTER_BOUND ( 'NONE', #34746, .T. ) ;
#29705=ORIENTED_EDGE ( 'NONE', *, *, #58762, .T. ) ;
#29706=DIRECTION ( 'NONE',  ( 0.000000000000000000, 0.000000000000000000, 1.000000000000000000 ) ) ;
#29840=AXIS2_PLACEMENT_3D ( 'NONE', #22124, #55172, #49536 ) ;
#29928=DIRECTION ( 'NONE',  ( 1.000000000000000000, 0.000000000000000000, 0.000000000000000000 ) ) ;
#29934=ORIENTED_EDGE ( 'NONE', *, *, #47858, .F. ) ;
#29975=ORIENTED_EDGE ( 'NONE', *, *, #1262, .T. ) ;
#30259=VERTEX_POINT ( 'NONE', #26476 ) ;
#30392=LINE ( 'NONE', #56089, #10051 ) ;
#30529=VERTEX_POINT ( 'NONE', #27069 ) ;
#30589=DIRECTION ( 'NONE',  ( 1.000000000000000000, 0.000000000000000000, -0.000000000000000000 ) ) ;
#30600=ORIENTED_EDGE ( 'NONE', *, *, #8624, .F. ) ;
#30612=ADVANCED_FACE ( 'NONE', ( #65776 ), #33058, .T. ) ;
#30651=VECTOR ( 'NONE', #18029, 1000.000000000000000 ) ;
#30662=VERTEX_POINT ( 'NONE', #59765 ) ;
#30849=AXIS2_PLACEMENT_3D ( 'NONE', #34050, #55855, #2049 ) ;
#31057=DIRECTION ( 'NONE',  ( 0.000000000000000000, 0.000000000000000000, 1.000000000000000000 ) ) ;
#31064=CARTESIAN_POINT ( 'NONE',  ( -89.99999999999998579, 1.102182119232617596E-14, -10.00000000000000000 ) ) ;
#31115=AXIS2_PLACEMENT_3D ( 'NONE', #61213, #41146, #7758 ) ;
#31291=CIRCLE ( 'NONE', #7697, 89.99999999999998579 ) ;
#31317=DIRECTION ( 'NONE',  ( -0.000000000000000000, -0.000000000000000000, 1.000000000000000000 ) ) ;
#31345=DIRECTION ( 'NONE',  ( 0.9561276726666719794, 0.000000000000000000, 0.2929502919626694180 ) ) ;
#31449=DIRECTION ( 'NONE',  ( -0.000000000000000000, -0.000000000000000000, 1.000000000000000000 ) ) ;
#31458=AXIS2_PLACEMENT_3D ( 'NONE', #65119, #53842, #27826 ) ;
#31571=CIRCLE ( 'NONE', #20321, 10.00000000000000178 ) ;
#31576=CARTESIAN_POINT ( 'NONE',  ( -89.99999999999998579, 1.102182119232617596E-14, 10.00000000000000000 ) ) ;
#31582=EDGE_LOOP ( 'NONE', ( #29934, #24087, #62521, #48621 ) ) ;
#31637=DIRECTION ( 'NONE',  ( -0.000000000000000000, -0.000000000000000000, -1.000000000000000000 ) ) ;
#31643=DIRECTION ( 'NONE',  ( -0.000000000000000000, -0.000000000000000000, -1.000000000000000000 ) ) ;
#31842=CIRCLE ( 'NONE', #49808, 10.00000000000000000 ) ;
#31849=DIRECTION ( 'NONE',  ( 0.000000000000000000, 0.000000000000000000, 1.000000000000000000 ) ) ;
#31988=FACE_OUTER_BOUND ( 'NONE', #2431, .T. ) ;
#32295=CIRCLE ( 'NONE', #49134, 10.00000000000000178 ) ;
#32354=DIRECTION ( 'NONE',  ( -0.000000000000000000, -0.000000000000000000, 1.000000000000000000 ) ) ;
#32508=CYLINDRICAL_SURFACE ( 'NONE', #21446, 89.99999999999998579 ) ;
#32524=CARTESIAN_POINT ( 'NONE',  ( 45.39413431650373809, 0.000000000000000000, 5.000000000000000000 ) ) ;
#32638=DIRECTION ( 'NONE',  ( -0.000000000000000000, -0.000000000000000000, 1.000000000000000000 ) ) ;
#32933=DIRECTION ( 'NONE',  ( -0.000000000000000000, -0.000000000000000000, 1.000000000000000000 ) ) ;
#32956=DIRECTION ( 'NONE',  ( -1.000000000000000000, 0.000000000000000000, 0.000000000000000000 ) ) ;
#33023=DIRECTION ( 'NONE',  ( 1.000000000000000000, 0.000000000000000000, 0.000000000000000000 ) ) ;
#33031=DIRECTION ( 'NONE',  ( 0.000000000000000000, 0.000000000000000000, 1.000000000000000000 ) ) ;
#33058=CYLINDRICAL_SURFACE ( 'NONE', #6486, 89.99999999999998579 ) ;
#33067=CIRCLE ( 'NONE', #2740, 10.00000000000000178 ) ;
#33068=ORIENTED_EDGE ( 'NONE', *, *, #38565, .F. ) ;
#33076=DIRECTION ( 'NONE',  ( 1.000000000000000000, 0.000000000000000000, 0.000000000000000000 ) ) ;
#33142=EDGE_CURVE ( 'NONE', #28536, #30662, #36815, .T. ) ;
#33206=ORIENTED_EDGE ( 'NONE', *, *, #7463, .F. ) ;
#33419=EDGE_CURVE ( 'NONE', #21145, #18591, #46234, .T. ) ;
#33560=DIRECTION ( 'NONE',  ( 0.000000000000000000, 0.000000000000000000, -1.000000000000000000 ) ) ;
#33604=ORIENTED_EDGE ( 'NONE', *, *, #14075, .F. ) ;
#33611=CIRCLE ( 'NONE', #49291, 89.99999999999998579 ) ;
#33731=CYLINDRICAL_SURFACE ( 'NONE', #59053, 10.00000000000000178 ) ;
#33842=DIRECTION ( 'NONE',  ( -1.000000000000000000, 0.000000000000000000, 0.000000000000000000 ) ) ;
#33872=CARTESIAN_POINT ( 'NONE',  ( 0.000000000000000000, 0.000000000000000000, 0.000000000000000000 ) ) ;
#34011=CARTESIAN_POINT ( 'NONE',  ( -34.39004539972345498, 0.000000000000000000, -9.999999999999998224 ) ) ;
#34037=CYLINDRICAL_SURFACE ( 'NONE', #37303, 10.00000000000000178 ) ;
#34050=CARTESIAN_POINT ( 'NONE',  ( 35.39413431650373099, 0.000000000000000000, -9.999999999999998224 ) ) ;
#34089=CARTESIAN_POINT ( 'NONE',  ( 60.00000000000000000, 7.347880794884118356E-15, -5.000000000000000000 ) ) ;
#34171=STYLED_ITEM ( 'NONE', ( #12653 ), #41867 ) ;
#34312=EDGE_CURVE ( 'NONE', #65175, #10742, #22413, .T. ) ;
#34386=VECTOR ( 'NONE', #31345, 1000.000000000000227 ) ;
#34420=DIRECTION ( 'NONE',  ( 0.000000000000000000, 0.000000000000000000, -1.000000000000000000 ) ) ;
#34452=ORIENTED_EDGE ( 'NONE', *, *, #58933, .F. ) ;
#34616=CARTESIAN_POINT ( 'NONE',  ( 0.000000000000000000, 0.000000000000000000, -5.000000000000000000 ) ) ;
#34740=ADVANCED_FACE ( 'NONE', ( #53502 ), #21846, .T. ) ;
#34746=EDGE_LOOP ( 'NONE', ( #34945, #42625 ) ) ;
#34780=CARTESIAN_POINT ( 'NONE',  ( -10.00000000000000178, 35.26862320190615208, 5.000000000000000000 ) ) ;
#34832=DIRECTION ( 'NONE',  ( 1.000000000000000000, 0.000000000000000000, 0.000000000000000000 ) ) ;
#34887=ORIENTED_EDGE ( 'NONE', *, *, #48732, .F. ) ;
#34944=ORIENTED_EDGE ( 'NONE', *, *, #47265, .F. ) ;
#34945=ORIENTED_EDGE ( 'NONE', *, *, #19013, .T. ) ;
#35132=AXIS2_PLACEMENT_3D ( 'NONE', #6834, #53952, #11757 ) ;
#35304=CARTESIAN_POINT ( 'NONE',  ( -34.39004539972345498, 0.000000000000000000, -5.000000000000000000 ) ) ;
#35433=ADVANCED_FACE ( 'NONE', ( #56556 ), #62177, .F. ) ;
#35438=FACE_OUTER_BOUND ( 'NONE', #68611, .T. ) ;
#35449=CARTESIAN_POINT ( 'NONE',  ( -24.39004539972345498, 0.000000000000000000, -5.000000000000000000 ) ) ;
#35485=AXIS2_PLACEMENT_3D ( 'NONE', #10178, #47810, #59397 ) ;
#35525=CYLINDRICAL_SURFACE ( 'NONE', #31115, 75.31295361348102801 ) ;
#35656=DIRECTION ( 'NONE',  ( -1.000000000000000000, 0.000000000000000000, 0.000000000000000000 ) ) ;
#35668=AXIS2_PLACEMENT_3D ( 'NONE', #60901, #65493, #7453 ) ;
#35837=ORIENTED_EDGE ( 'NONE', *, *, #63523, .F. ) ;
#35850=DIRECTION ( 'NONE',  ( -0.000000000000000000, -0.000000000000000000, 1.000000000000000000 ) ) ;
#35900=ADVANCED_FACE ( 'NONE', ( #44810 ), #32508, .T. ) ;
#35937=ORIENTED_EDGE ( 'NONE', *, *, #25747, .T. ) ;
#36062=DIRECTION ( 'NONE',  ( -1.000000000000000000, 0.000000000000000000, 0.000000000000000000 ) ) ;
#36283=AXIS2_PLACEMENT_3D ( 'NONE', #34011, #54394, #22054 ) ;
#36345=( LENGTH_UNIT ( ) NAMED_UNIT ( * ) SI_UNIT ( .MILLI., .METRE. ) );
#36395=CARTESIAN_POINT ( 'NONE',  ( -10.00000000000000178, -31.50328976398030534, 5.000000000000000000 ) ) ;
#36436=ORIENTED_EDGE ( 'NONE', *, *, #51736, .T. ) ;
#36631=PRODUCT_DEFINITION_FORMATION_WITH_SPECIFIED_SOURCE ( 'ANY', '', #52880, .NOT_KNOWN. ) ;
#36753=DIRECTION ( 'NONE',  ( 0.000000000000000000, 0.000000000000000000, -1.000000000000000000 ) ) ;
#36765=AXIS2_PLACEMENT_3D ( 'NONE', #18687, #2167, #23619 ) ;
#36807=DIRECTION ( 'NONE',  ( -1.000000000000000000, 0.000000000000000000, 0.000000000000000000 ) ) ;
#36815=LINE ( 'NONE', #13374, #22395 ) ;
#36979=ORIENTED_EDGE ( 'NONE', *, *, #19586, .T. ) ;
#37249=FACE_BOUND ( 'NONE', #55559, .T. ) ;
#37303=AXIS2_PLACEMENT_3D ( 'NONE', #12934, #55839, #61457 ) ;
#37511=CIRCLE ( 'NONE', #38626, 89.99999999999998579 ) ;
#37542=PLANE ( 'NONE',  #55804 ) ;
#37562=CYLINDRICAL_SURFACE ( 'NONE', #62671, 60.00000000000000000 ) ;
#37622=CIRCLE ( 'NONE', #7317, 89.99999999999998579 ) ;
#37697=CARTESIAN_POINT ( 'NONE',  ( 0.000000000000000000, 0.000000000000000000, 10.00000000000000000 ) ) ;
#37847=ORIENTED_EDGE ( 'NONE', *, *, #65020, .T. ) ;
#37948=FACE_BOUND ( 'NONE', #61800, .T. ) ;
#37950=VECTOR ( 'NONE', #59935, 1000.000000000000000 ) ;
#38081=EDGE_LOOP ( 'NONE', ( #54629, #58652, #68148, #11681 ) ) ;
#38115=DIRECTION ( 'NONE',  ( 1.000000000000000000, 0.000000000000000000, 0.000000000000000000 ) ) ;
#38134=APPLICATION_CONTEXT ( 'automotive_design' ) ;
#38245=CARTESIAN_POINT ( 'NONE',  ( 0.000000000000000000, 0.000000000000000000, -7.000000000000000000 ) ) ;
#38498=CARTESIAN_POINT ( 'NONE',  ( 10.00000000000000178, 35.26862320190615208, 5.000000000000000000 ) ) ;
#38501=ADVANCED_FACE ( 'NONE', ( #39655 ), #34037, .F. ) ;
#38565=EDGE_CURVE ( 'NONE', #43150, #10057, #56405, .T. ) ;
#38626=AXIS2_PLACEMENT_3D ( 'NONE', #25871, #4067, #25533 ) ;
#38754=DIRECTION ( 'NONE',  ( -0.000000000000000000, -0.000000000000000000, 1.000000000000000000 ) ) ;
#38790=EDGE_CURVE ( 'NONE', #9869, #68905, #24000, .T. ) ;
#39009=CARTESIAN_POINT ( 'NONE',  ( 0.000000000000000000, 35.26862320190615208, -9.999999999999998224 ) ) ;
#39063=ORIENTED_EDGE ( 'NONE', *, *, #4704, .T. ) ;
#39133=EDGE_LOOP ( 'NONE', ( #45024, #7333 ) ) ;
#39170=VERTEX_POINT ( 'NONE', #43126 ) ;
#39364=LINE ( 'NONE', #48490, #40856 ) ;
#39394=CARTESIAN_POINT ( 'NONE',  ( 0.000000000000000000, 0.000000000000000000, 10.00000000000000000 ) ) ;
#39594=CARTESIAN_POINT ( 'NONE',  ( 0.000000000000000000, 35.26862320190615208, 5.000000000000000000 ) ) ;
#39655=FACE_OUTER_BOUND ( 'NONE', #52021, .T. ) ;
#39660=ORIENTED_EDGE ( 'NONE', *, *, #33419, .F. ) ;
#39743=ORIENTED_EDGE ( 'NONE', *, *, #1694, .T. ) ;
#39768=EDGE_LOOP ( 'NONE', ( #51397, #9685, #23675, #26119 ) ) ;
#39998=VERTEX_POINT ( 'NONE', #34780 ) ;
#40035=DIRECTION ( 'NONE',  ( 0.000000000000000000, 0.000000000000000000, -1.000000000000000000 ) ) ;
#40042=ORIENTED_EDGE ( 'NONE', *, *, #66502, .F. ) ;
#40227=ORIENTED_EDGE ( 'NONE', *, *, #64054, .T. ) ;
#40242=SHAPE_REPRESENTATION_RELATIONSHIP ( 'NONE' , 'NONE' ,  #7414, #56683 ) ;
#40347=EDGE_CURVE ( 'NONE', #21319, #52293, #59948, .T. ) ;
#40362=ADVANCED_FACE ( 'NONE', ( #69099 ), #50988, .T. ) ;
#40595=DIRECTION ( 'NONE',  ( -0.000000000000000000, -0.000000000000000000, 1.000000000000000000 ) ) ;
#40785=PLANE ( 'NONE',  #57376 ) ;
#40805=CARTESIAN_POINT ( 'NONE',  ( 10.00000000000000000, 0.000000000000000000, 5.000000000000000000 ) ) ;
#40856=VECTOR ( 'NONE', #32354, 1000.000000000000000 ) ;
#40976=DIRECTION ( 'NONE',  ( 1.000000000000000000, 0.000000000000000000, 0.000000000000000000 ) ) ;
#41042=EDGE_CURVE ( 'NONE', #27439, #6794, #53262, .T. ) ;
#41146=DIRECTION ( 'NONE',  ( -0.000000000000000000, -0.000000000000000000, 1.000000000000000000 ) ) ;
#41147=VECTOR ( 'NONE', #19525, 1000.000000000000000 ) ;
#41564=AXIS2_PLACEMENT_3D ( 'NONE', #5081, #58205, #26547 ) ;
#41619=( NAMED_UNIT ( * ) PLANE_ANGLE_UNIT ( ) SI_UNIT ( $, .RADIAN. ) );
#41632=EDGE_CURVE ( 'NONE', #50425, #56268, #31842, .T. ) ;
#41751=AXIS2_PLACEMENT_3D ( 'NONE', #45973, #62851, #67441 ) ;
#41856=LINE ( 'NONE', #57344, #3589 ) ;
#41857=VECTOR ( 'NONE', #15564, 1000.000000000000000 ) ;
#41867=MANIFOLD_SOLID_BREP ( 'Cut-Revolve1', #66543 ) ;
#42035=DIRECTION ( 'NONE',  ( 0.000000000000000000, 0.000000000000000000, -1.000000000000000000 ) ) ;
#42134=FACE_BOUND ( 'NONE', #45311, .T. ) ;
#42136=AXIS2_PLACEMENT_3D ( 'NONE', #44076, #33560, #15971 ) ;
#42146=DIRECTION ( 'NONE',  ( -0.000000000000000000, -0.000000000000000000, 1.000000000000000000 ) ) ;
#42150=AXIS2_PLACEMENT_3D ( 'NONE', #33872, #60945, #11354 ) ;
#42161=ORIENTED_EDGE ( 'NONE', *, *, #58762, .F. ) ;
#42299=DIRECTION ( 'NONE',  ( 0.000000000000000000, 0.000000000000000000, 1.000000000000000000 ) ) ;
#42324=LINE ( 'NONE', #59174, #4888 ) ;
#42345=AXIS2_PLACEMENT_3D ( 'NONE', #20066, #9510, #29928 ) ;
#42473=ADVANCED_FACE ( 'NONE', ( #35438 ), #67797, .F. ) ;
#42538=FACE_BOUND ( 'NONE', #28623, .T. ) ;
#42625=ORIENTED_EDGE ( 'NONE', *, *, #2236, .T. ) ;
#42732=DIRECTION ( 'NONE',  ( 0.000000000000000000, 0.000000000000000000, -1.000000000000000000 ) ) ;
#42910=CARTESIAN_POINT ( 'NONE',  ( 75.31295361348104223, 9.223176757708265897E-15, -2.499999999999970246 ) ) ;
#42997=EDGE_LOOP ( 'NONE', ( #16580, #6243, #69449, #55082 ) ) ;
#43060=DIRECTION ( 'NONE',  ( -0.000000000000000000, -0.000000000000000000, 1.000000000000000000 ) ) ;
#43098=AXIS2_PLACEMENT_3D ( 'NONE', #37697, #42299, #5354 ) ;
#43103=ORIENTED_EDGE ( 'NONE', *, *, #33142, .T. ) ;
#43122=ORIENTED_EDGE ( 'NONE', *, *, #20955, .T. ) ;
#43126=CARTESIAN_POINT ( 'NONE',  ( 45.39413431650373809, 0.000000000000000000, -5.000000000000000000 ) ) ;
#43150=VERTEX_POINT ( 'NONE', #18919 ) ;
#43562=ADVANCED_FACE ( 'NONE', ( #22637 ), #18587, .T. ) ;
#43943=CIRCLE ( 'NONE', #60832, 10.00000000000000178 ) ;
#44007=CONICAL_SURFACE ( 'NONE', #52987, 89.99999999999998579, 1.273485274044415583 ) ;
#44012=EDGE_LOOP ( 'NONE', ( #13196, #46588 ) ) ;
#44076=CARTESIAN_POINT ( 'NONE',  ( 0.000000000000000000, 0.000000000000000000, -2.499999999999970246 ) ) ;
#44086=CIRCLE ( 'NONE', #17125, 10.00000000000000178 ) ;
#44091=ORIENTED_EDGE ( 'NONE', *, *, #47160, .F. ) ;
#44097=AXIS2_PLACEMENT_3D ( 'NONE', #5011, #63768, #21198 ) ;
#44184=AXIS2_PLACEMENT_3D ( 'NONE', #34616, #31643, #24744 ) ;
#44200=ORIENTED_EDGE ( 'NONE', *, *, #38565, .T. ) ;
#44339=CONICAL_SURFACE ( 'NONE', #2793, 89.99999999999998579, 1.273485274044415583 ) ;
#44416=CYLINDRICAL_SURFACE ( 'NONE', #42150, 75.31295361348102801 ) ;
#44441=EDGE_LOOP ( 'NONE', ( #12106, #27547, #29705, #34887 ) ) ;
#44558=DIRECTION ( 'NONE',  ( 0.000000000000000000, 0.000000000000000000, 1.000000000000000000 ) ) ;
#44600=ORIENTED_EDGE ( 'NONE', *, *, #27949, .T. ) ;
#44810=FACE_OUTER_BOUND ( 'NONE', #4769, .T. ) ;
#44947=VERTEX_POINT ( 'NONE', #21581 ) ;
#45024=ORIENTED_EDGE ( 'NONE', *, *, #4914, .F. ) ;
#45232=EDGE_LOOP ( 'NONE', ( #58020, #34944 ) ) ;
#45239=DIRECTION ( 'NONE',  ( -0.000000000000000000, -0.000000000000000000, 1.000000000000000000 ) ) ;
#45311=EDGE_LOOP ( 'NONE', ( #48689, #8682 ) ) ;
#45321=DIRECTION ( 'NONE',  ( -0.000000000000000000, -0.000000000000000000, -1.000000000000000000 ) ) ;
#45322=DIRECTION ( 'NONE',  ( -0.000000000000000000, -0.000000000000000000, 1.000000000000000000 ) ) ;
#45363=VERTEX_POINT ( 'NONE', #53841 ) ;
#45420=DIRECTION ( 'NONE',  ( -1.000000000000000000, 0.000000000000000000, 0.000000000000000000 ) ) ;
#45430=CARTESIAN_POINT ( 'NONE',  ( 0.000000000000000000, 0.000000000000000000, -4.999999999999997335 ) ) ;
#45455=CARTESIAN_POINT ( 'NONE',  ( 0.000000000000000000, 0.000000000000000000, -10.00000000000000000 ) ) ;
#45465=CARTESIAN_POINT ( 'NONE',  ( 0.000000000000000000, 0.000000000000000000, 5.000000000000000000 ) ) ;
#45537=CARTESIAN_POINT ( 'NONE',  ( 10.00000000000000000, 0.000000000000000000, -4.999999999999997335 ) ) ;
#45801=EDGE_LOOP ( 'NONE', ( #68335, #36979, #35937, #3553 ) ) ;
#45859=CIRCLE ( 'NONE', #16619, 10.00000000000000178 ) ;
#45973=CARTESIAN_POINT ( 'NONE',  ( 0.000000000000000000, 0.000000000000000000, 5.000000000000000000 ) ) ;
#46234=LINE ( 'NONE', #9299, #13464 ) ;
#46295=EDGE_LOOP ( 'NONE', ( #61392, #8935, #5069, #44091 ) ) ;
#46300=EDGE_CURVE ( 'NONE', #68618, #61781, #15212, .T. ) ;
#46312=ORIENTED_EDGE ( 'NONE', *, *, #2163, .T. ) ;
#46538=EDGE_CURVE ( 'NONE', #18591, #2403, #13176, .T. ) ;
#46543=( NAMED_UNIT ( * ) SI_UNIT ( $, .STERADIAN. ) SOLID_ANGLE_UNIT ( ) );
#46588=ORIENTED_EDGE ( 'NONE', *, *, #64406, .F. ) ;
#46751=AXIS2_PLACEMENT_3D ( 'NONE', #59740, #33031, #60098 ) ;
#47066=DIRECTION ( 'NONE',  ( 0.000000000000000000, 0.000000000000000000, -1.000000000000000000 ) ) ;
#47098=ORIENTED_EDGE ( 'NONE', *, *, #27892, .F. ) ;
#47138=ORIENTED_EDGE ( 'NONE', *, *, #4897, .T. ) ;
#47160=EDGE_CURVE ( 'NONE', #9547, #56182, #26666, .T. ) ;
#47265=EDGE_CURVE ( 'NONE', #22725, #39170, #32295, .T. ) ;
#47374=ADVANCED_FACE ( 'NONE', ( #12372 ), #49998, .F. ) ;
#47375=ORIENTED_EDGE ( 'NONE', *, *, #19527, .F. ) ;
#47396=DIRECTION ( 'NONE',  ( 1.000000000000000000, 0.000000000000000000, 0.000000000000000000 ) ) ;
#47554=VECTOR ( 'NONE', #54794, 999.9999999999998863 ) ;
#47684=VERTEX_POINT ( 'NONE', #28018 ) ;
#47810=DIRECTION ( 'NONE',  ( 0.000000000000000000, 0.000000000000000000, 1.000000000000000000 ) ) ;
#47815=CYLINDRICAL_SURFACE ( 'NONE', #44184, 60.00000000000000000 ) ;
#47858=EDGE_CURVE ( 'NONE', #56268, #30529, #58897, .T. ) ;
#47864=EDGE_CURVE ( 'NONE', #66948, #53100, #10712, .T. ) ;
#47957=DIRECTION ( 'NONE',  ( 1.000000000000000000, 0.000000000000000000, 0.000000000000000000 ) ) ;
#48031=VECTOR ( 'NONE', #43060, 1000.000000000000000 ) ;
#48184=LINE ( 'NONE', #42910, #5982 ) ;
#48449=AXIS2_PLACEMENT_3D ( 'NONE', #58038, #31317, #53083 ) ;
#48460=ORIENTED_EDGE ( 'NONE', *, *, #4704, .F. ) ;
#48490=CARTESIAN_POINT ( 'NONE',  ( -75.31295361348102801, 9.223176757708264319E-15, 0.000000000000000000 ) ) ;
#48576=ORIENTED_EDGE ( 'NONE', *, *, #7236, .T. ) ;
#48592=DIRECTION ( 'NONE',  ( -0.000000000000000000, -0.000000000000000000, 1.000000000000000000 ) ) ;
#48621=ORIENTED_EDGE ( 'NONE', *, *, #19463, .T. ) ;
#48689=ORIENTED_EDGE ( 'NONE', *, *, #16244, .F. ) ;
#48732=EDGE_CURVE ( 'NONE', #68905, #13402, #31291, .T. ) ;
#49079=DIRECTION ( 'NONE',  ( 1.000000000000000000, 0.000000000000000000, 0.000000000000000000 ) ) ;
#49134=AXIS2_PLACEMENT_3D ( 'NONE', #17290, #60556, #45420 ) ;
#49156=CARTESIAN_POINT ( 'NONE',  ( -75.31295361348104223, 0.000000000000000000, -2.499999999999970246 ) ) ;
#49194=ORIENTED_EDGE ( 'NONE', *, *, #27949, .F. ) ;
#49224=ORIENTED_EDGE ( 'NONE', *, *, #56684, .F. ) ;
#49291=AXIS2_PLACEMENT_3D ( 'NONE', #45455, #67288, #2555 ) ;
#49377=VECTOR ( 'NONE', #32933, 1000.000000000000000 ) ;
#49508=CARTESIAN_POINT ( 'NONE',  ( 60.00000000000000000, 7.347880794884118356E-15, -10.00000000000000000 ) ) ;
#49536=DIRECTION ( 'NONE',  ( 1.000000000000000000, 0.000000000000000000, 0.000000000000000000 ) ) ;
#49679=FACE_OUTER_BOUND ( 'NONE', #38081, .T. ) ;
#49690=EDGE_CURVE ( 'NONE', #65175, #52293, #13697, .T. ) ;
#49749=ORIENTED_EDGE ( 'NONE', *, *, #52805, .T. ) ;
#49808=AXIS2_PLACEMENT_3D ( 'NONE', #45430, #23979, #33842 ) ;
#49864=ADVANCED_FACE ( 'NONE', ( #63954 ), #37562, .F. ) ;
#49932=CARTESIAN_POINT ( 'NONE',  ( -44.39004539972346208, 1.224646799147353256E-15, -9.999999999999998224 ) ) ;
#49984=AXIS2_PLACEMENT_3D ( 'NONE', #64145, #474, #47957 ) ;
#49998=CYLINDRICAL_SURFACE ( 'NONE', #35668, 60.00000000000000000 ) ;
#50034=CIRCLE ( 'NONE', #54528, 60.00000000000000000 ) ;
#50090=CARTESIAN_POINT ( 'NONE',  ( 10.00000000000000178, -31.50328976398030534, -5.000000000000000000 ) ) ;
#50259=DIRECTION ( 'NONE',  ( 1.000000000000000000, 0.000000000000000000, 0.000000000000000000 ) ) ;
#50308=FACE_OUTER_BOUND ( 'NONE', #21868, .T. ) ;
#50425=VERTEX_POINT ( 'NONE', #45537 ) ;
#50530=CARTESIAN_POINT ( 'NONE',  ( 0.000000000000000000, 0.000000000000000000, 0.000000000000000000 ) ) ;
#50794=CIRCLE ( 'NONE', #26047, 89.99999999999998579 ) ;
#50934=DIRECTION ( 'NONE',  ( 0.000000000000000000, 0.000000000000000000, -1.000000000000000000 ) ) ;
#50988=CONICAL_SURFACE ( 'NONE', #64479, 75.31295361348104223, 1.273485274044411586 ) ;
#51280=VECTOR ( 'NONE', #31057, 1000.000000000000000 ) ;
#51360=FACE_OUTER_BOUND ( 'NONE', #42997, .T. ) ;
#51397=ORIENTED_EDGE ( 'NONE', *, *, #12100, .T. ) ;
#51545=ADVANCED_FACE ( 'NONE', ( #13049 ), #23251, .F. ) ;
#51700=EDGE_CURVE ( 'NONE', #30529, #20755, #25997, .T. ) ;
#51736=EDGE_CURVE ( 'NONE', #53637, #30259, #43943, .T. ) ;
#51784=EDGE_CURVE ( 'NONE', #13402, #68905, #50794, .T. ) ;
#51849=CARTESIAN_POINT ( 'NONE',  ( 0.000000000000000000, -31.50328976398030534, 5.000000000000000000 ) ) ;
#51934=DIRECTION ( 'NONE',  ( 0.000000000000000000, 0.000000000000000000, 1.000000000000000000 ) ) ;
#52021=EDGE_LOOP ( 'NONE', ( #30600, #2790, #62447, #44200 ) ) ;
#52028=DIRECTION ( 'NONE',  ( 1.000000000000000000, 0.000000000000000000, 0.000000000000000000 ) ) ;
#52054=DIRECTION ( 'NONE',  ( -0.000000000000000000, -0.000000000000000000, 1.000000000000000000 ) ) ;
#52293=VERTEX_POINT ( 'NONE', #7775 ) ;
#52323=EDGE_CURVE ( 'NONE', #2893, #56182, #41856, .T. ) ;
#52348=FACE_BOUND ( 'NONE', #44012, .T. ) ;
#52613=ORIENTED_EDGE ( 'NONE', *, *, #8624, .T. ) ;
#52680=FACE_BOUND ( 'NONE', #28936, .T. ) ;
#52805=EDGE_CURVE ( 'NONE', #22725, #30259, #6559, .T. ) ;
#52828=CARTESIAN_POINT ( 'NONE',  ( 89.99999999999998579, 0.000000000000000000, -10.00000000000000000 ) ) ;
#52841=FACE_BOUND ( 'NONE', #20358, .T. ) ;
#52880=PRODUCT ( 'pulley', 'pulley', '', ( #67767 ) ) ;
#52987=AXIS2_PLACEMENT_3D ( 'NONE', #62933, #14735, #52028 ) ;
#53030=DIRECTION ( 'NONE',  ( 1.000000000000000000, 0.000000000000000000, 0.000000000000000000 ) ) ;
#53083=DIRECTION ( 'NONE',  ( 1.000000000000000000, 0.000000000000000000, 0.000000000000000000 ) ) ;
#53100=VERTEX_POINT ( 'NONE', #68190 ) ;
#53211=VERTEX_POINT ( 'NONE', #31576 ) ;
#53262=CIRCLE ( 'NONE', #22964, 10.00000000000000178 ) ;
#53321=ADVANCED_FACE ( 'NONE', ( #12551 ), #6575, .F. ) ;
#53502=FACE_OUTER_BOUND ( 'NONE', #44441, .T. ) ;
#53569=AXIS2_PLACEMENT_3D ( 'NONE', #12276, #45322, #50259 ) ;
#53637=VERTEX_POINT ( 'NONE', #32524 ) ;
#53650=DIRECTION ( 'NONE',  ( 1.000000000000000000, 0.000000000000000000, 0.000000000000000000 ) ) ;
#53655=ADVANCED_FACE ( 'NONE', ( #17382 ), #55013, .F. ) ;
#53841=CARTESIAN_POINT ( 'NONE',  ( 89.99999999999998579, 0.000000000000000000, -10.00000000000000000 ) ) ;
#53842=DIRECTION ( 'NONE',  ( 0.000000000000000000, 0.000000000000000000, 1.000000000000000000 ) ) ;
#53950=CARTESIAN_POINT ( 'NONE',  ( 75.31295361348102801, 0.000000000000000000, 0.000000000000000000 ) ) ;
#53952=DIRECTION ( 'NONE',  ( -0.000000000000000000, -0.000000000000000000, 1.000000000000000000 ) ) ;
#54063=DIRECTION ( 'NONE',  ( 1.000000000000000000, 0.000000000000000000, 0.000000000000000000 ) ) ;
#54082=CIRCLE ( 'NONE', #48449, 75.31295361348104223 ) ;
#54394=DIRECTION ( 'NONE',  ( -0.000000000000000000, -0.000000000000000000, 1.000000000000000000 ) ) ;
#54520=ORIENTED_EDGE ( 'NONE', *, *, #65020, .F. ) ;
#54528=AXIS2_PLACEMENT_3D ( 'NONE', #45465, #19778, #24720 ) ;
#54629=ORIENTED_EDGE ( 'NONE', *, *, #16686, .T. ) ;
#54794=DIRECTION ( 'NONE',  ( -0.9561276726666709802, 0.000000000000000000, -0.2929502919626733037 ) ) ;
#54806=CARTESIAN_POINT ( 'NONE',  ( 35.39413431650373099, 0.000000000000000000, -5.000000000000000000 ) ) ;
#55005=UNCERTAINTY_MEASURE_WITH_UNIT (LENGTH_MEASURE( 1.000000000000000082E-05 ), #55200, 'distance_accuracy_value', 'NONE');
#55013=CYLINDRICAL_SURFACE ( 'NONE', #35132, 10.00000000000000178 ) ;
#55082=ORIENTED_EDGE ( 'NONE', *, *, #19586, .F. ) ;
#55083=CARTESIAN_POINT ( 'NONE',  ( -10.00000000000000178, -31.50328976398030534, -9.999999999999998224 ) ) ;
#55172=DIRECTION ( 'NONE',  ( -0.000000000000000000, -0.000000000000000000, 1.000000000000000000 ) ) ;
#55200=( LENGTH_UNIT ( ) NAMED_UNIT ( * ) SI_UNIT ( .MILLI., .METRE. ) );
#55334=DIRECTION ( 'NONE',  ( -0.000000000000000000, -0.000000000000000000, 1.000000000000000000 ) ) ;
#55559=EDGE_LOOP ( 'NONE', ( #21136, #16620 ) ) ;
#55652=EDGE_CURVE ( 'NONE', #10057, #43150, #33067, .T. ) ;
#55690=CARTESIAN_POINT ( 'NONE',  ( -10.00000000000000178, 35.26862320190615208, -9.999999999999998224 ) ) ;
#55716=APPLICATION_CONTEXT ( 'automotive_design' ) ;
#55804=AXIS2_PLACEMENT_3D ( 'NONE', #3816, #47066, #47396 ) ;
#55839=DIRECTION ( 'NONE',  ( -0.000000000000000000, -0.000000000000000000, 1.000000000000000000 ) ) ;
#55846=ORIENTED_EDGE ( 'NONE', *, *, #58933, .T. ) ;
#55855=DIRECTION ( 'NONE',  ( -0.000000000000000000, -0.000000000000000000, 1.000000000000000000 ) ) ;
#55890=VECTOR ( 'NONE', #35850, 1000.000000000000000 ) ;
#55952=LINE ( 'NONE', #13724, #18616 ) ;
#56089=CARTESIAN_POINT ( 'NONE',  ( 10.00000000000000178, 35.26862320190615208, -9.999999999999998224 ) ) ;
#56182=VERTEX_POINT ( 'NONE', #2428 ) ;
#56205=CARTESIAN_POINT ( 'NONE',  ( 0.000000000000000000, 0.000000000000000000, -4.999999999999997335 ) ) ;
#56268=VERTEX_POINT ( 'NONE', #24873 ) ;
#56388=ADVANCED_FACE ( 'NONE', ( #15691 ), #14996, .F. ) ;
#56405=CIRCLE ( 'NONE', #14817, 10.00000000000000178 ) ;
#56429=ORIENTED_EDGE ( 'NONE', *, *, #4914, .T. ) ;
#56472=AXIS2_PLACEMENT_3D ( 'NONE', #60278, #59559, #38115 ) ;
#56556=FACE_OUTER_BOUND ( 'NONE', #22787, .T. ) ;
#56567=AXIS2_PLACEMENT_3D ( 'NONE', #39394, #6334, #33076 ) ;
#56605=AXIS2_PLACEMENT_3D ( 'NONE', #63152, #9689, #14612 ) ;
#56683=ADVANCED_BREP_SHAPE_REPRESENTATION ( '', ( #41867, #66832 ), #23071 ) ;
#56684=EDGE_CURVE ( 'NONE', #39170, #53637, #24106, .T. ) ;
#56700=ORIENTED_EDGE ( 'NONE', *, *, #56684, .T. ) ;
#56760=DIRECTION ( 'NONE',  ( 0.000000000000000000, 0.000000000000000000, -1.000000000000000000 ) ) ;
#56812=ORIENTED_EDGE ( 'NONE', *, *, #51784, .T. ) ;
#56880=ADVANCED_FACE ( 'NONE', ( #49679 ), #44416, .T. ) ;
#56979=FACE_BOUND ( 'NONE', #39133, .T. ) ;
#57091=CARTESIAN_POINT ( 'NONE',  ( -10.00000000000000178, 35.26862320190615208, -5.000000000000000000 ) ) ;
#57167=CARTESIAN_POINT ( 'NONE',  ( 89.99999999999998579, 0.000000000000000000, -10.00000000000000000 ) ) ;
#57321=ORIENTED_EDGE ( 'NONE', *, *, #51700, .T. ) ;
#57344=CARTESIAN_POINT ( 'NONE',  ( -60.00000000000000000, 0.000000000000000000, -5.000000000000000000 ) ) ;
#57376=AXIS2_PLACEMENT_3D ( 'NONE', #18993, #19678, #30589 ) ;
#57469=CIRCLE ( 'NONE', #41751, 10.00000000000000000 ) ;
#57489=CARTESIAN_POINT ( 'NONE',  ( 45.39413431650373809, 0.000000000000000000, -9.999999999999998224 ) ) ;
#57531=CARTESIAN_POINT ( 'NONE',  ( 0.000000000000000000, 0.000000000000000000, -2.499999999999970246 ) ) ;
#57638=AXIS2_PLACEMENT_3D ( 'NONE', #12519, #65645, #28344 ) ;
#57716=PRODUCT_DEFINITION ( 'UNKNOWN', '', #36631, #15578 ) ;
#57904=ORIENTED_EDGE ( 'NONE', *, *, #12100, .F. ) ;
#58008=CARTESIAN_POINT ( 'NONE',  ( 75.31295361348104223, 1.012249897501722014E-14, -2.499999999999970246 ) ) ;
#58020=ORIENTED_EDGE ( 'NONE', *, *, #20955, .F. ) ;
#58038=CARTESIAN_POINT ( 'NONE',  ( 0.000000000000000000, 0.000000000000000000, -2.499999999999970246 ) ) ;
#58137=CARTESIAN_POINT ( 'NONE',  ( 25.39413431650373099, 1.224646799147353059E-15, -5.000000000000000000 ) ) ;
#58140=FACE_OUTER_BOUND ( 'NONE', #12617, .T. ) ;
#58147=FACE_OUTER_BOUND ( 'NONE', #45801, .T. ) ;
#58205=DIRECTION ( 'NONE',  ( -0.000000000000000000, -0.000000000000000000, 1.000000000000000000 ) ) ;
#58250=CARTESIAN_POINT ( 'NONE',  ( 0.000000000000000000, 0.000000000000000000, -2.499999999999970246 ) ) ;
#58564=DIRECTION ( 'NONE',  ( 1.000000000000000000, 0.000000000000000000, 0.000000000000000000 ) ) ;
#58574=ORIENTED_EDGE ( 'NONE', *, *, #51736, .F. ) ;
#58619=CARTESIAN_POINT ( 'NONE',  ( 10.00000000000000000, 0.000000000000000000, -50.00000000000000711 ) ) ;
#58652=ORIENTED_EDGE ( 'NONE', *, *, #2780, .T. ) ;
#58762=EDGE_CURVE ( 'NONE', #45363, #13402, #67726, .T. ) ;
#58814=PLANE ( 'NONE',  #44097 ) ;
#58860=CARTESIAN_POINT ( 'NONE',  ( 0.000000000000000000, 0.000000000000000000, 7.000000000000000000 ) ) ;
#58897=LINE ( 'NONE', #11059, #48031 ) ;
#58908=AXIS2_PLACEMENT_3D ( 'NONE', #1416, #7039, #34832 ) ;
#58933=EDGE_CURVE ( 'NONE', #27439, #39998, #1529, .T. ) ;
#59050=FACE_BOUND ( 'NONE', #12808, .T. ) ;
#59053=AXIS2_PLACEMENT_3D ( 'NONE', #39009, #61152, #33023 ) ;
#59174=CARTESIAN_POINT ( 'NONE',  ( -24.39004539972345498, 0.000000000000000000, -9.999999999999998224 ) ) ;
#59233=ORIENTED_EDGE ( 'NONE', *, *, #3121, .T. ) ;
#59359=CARTESIAN_POINT ( 'NONE',  ( 0.000000000000000000, 0.000000000000000000, 5.000000000000000000 ) ) ;
#59392=DIRECTION ( 'NONE',  ( -0.000000000000000000, -0.000000000000000000, 1.000000000000000000 ) ) ;
#59397=DIRECTION ( 'NONE',  ( 1.000000000000000000, 0.000000000000000000, -0.000000000000000000 ) ) ;
#59439=LINE ( 'NONE', #5630, #34386 ) ;
#59559=DIRECTION ( 'NONE',  ( 0.000000000000000000, 0.000000000000000000, 1.000000000000000000 ) ) ;
#59598=VECTOR ( 'NONE', #11950, 1000.000000000000000 ) ;
#59701=AXIS2_PLACEMENT_3D ( 'NONE', #4782, #64920, #53650 ) ;
#59740=CARTESIAN_POINT ( 'NONE',  ( 0.000000000000000000, 0.000000000000000000, 5.000000000000000000 ) ) ;
#59765=CARTESIAN_POINT ( 'NONE',  ( -89.99999999999998579, 1.102182119232617596E-14, 7.000000000000000000 ) ) ;
#59908=ORIENTED_EDGE ( 'NONE', *, *, #49690, .F. ) ;
#59915=CIRCLE ( 'NONE', #43098, 89.99999999999998579 ) ;
#59935=DIRECTION ( 'NONE',  ( -0.000000000000000000, -0.000000000000000000, 1.000000000000000000 ) ) ;
#59945=( GEOMETRIC_REPRESENTATION_CONTEXT ( 3 ) GLOBAL_UNCERTAINTY_ASSIGNED_CONTEXT ( ( #55005 ) ) GLOBAL_UNIT_ASSIGNED_CONTEXT ( ( #55200, #28475, #1394 ) ) REPRESENTATION_CONTEXT ( 'NONE', 'WORKASPACE' ) );
#59948=CIRCLE ( 'NONE', #56605, 10.00000000000000178 ) ;
#60027=CARTESIAN_POINT ( 'NONE',  ( 0.000000000000000000, 35.26862320190615208, -5.000000000000000000 ) ) ;
#60070=VECTOR ( 'NONE', #45321, 1000.000000000000000 ) ;
#60080=ORIENTED_EDGE ( 'NONE', *, *, #7053, .F. ) ;
#60098=DIRECTION ( 'NONE',  ( 1.000000000000000000, 0.000000000000000000, 0.000000000000000000 ) ) ;
#60236=DIRECTION ( 'NONE',  ( 1.000000000000000000, 0.000000000000000000, 0.000000000000000000 ) ) ;
#60278=CARTESIAN_POINT ( 'NONE',  ( 0.000000000000000000, 35.26862320190615208, 5.000000000000000000 ) ) ;
#60287=CARTESIAN_POINT ( 'NONE',  ( 0.000000000000000000, 0.000000000000000000, -10.00000000000000000 ) ) ;
#60306=EDGE_CURVE ( 'NONE', #12451, #11248, #13038, .T. ) ;
#60437=CARTESIAN_POINT ( 'NONE',  ( -34.39004539972345498, 0.000000000000000000, -5.000000000000000000 ) ) ;
#60511=AXIS2_PLACEMENT_3D ( 'NONE', #56205, #40035, #22810 ) ;
#60522=ORIENTED_EDGE ( 'NONE', *, *, #22471, .T. ) ;
#60556=DIRECTION ( 'NONE',  ( 0.000000000000000000, 0.000000000000000000, -1.000000000000000000 ) ) ;
#60764=ORIENTED_EDGE ( 'NONE', *, *, #25747, .F. ) ;
#60827=CIRCLE ( 'NONE', #59701, 75.31295361348102801 ) ;
#60832=AXIS2_PLACEMENT_3D ( 'NONE', #66355, #1261, #7241 ) ;
#60901=CARTESIAN_POINT ( 'NONE',  ( 0.000000000000000000, 0.000000000000000000, 5.000000000000000000 ) ) ;
#60933=CARTESIAN_POINT ( 'NONE',  ( -89.99999999999998579, 1.102182119232617596E-14, -10.00000000000000000 ) ) ;
#60945=DIRECTION ( 'NONE',  ( -0.000000000000000000, -0.000000000000000000, 1.000000000000000000 ) ) ;
#61152=DIRECTION ( 'NONE',  ( -0.000000000000000000, -0.000000000000000000, 1.000000000000000000 ) ) ;
#61213=CARTESIAN_POINT ( 'NONE',  ( 0.000000000000000000, 0.000000000000000000, 0.000000000000000000 ) ) ;
#61392=ORIENTED_EDGE ( 'NONE', *, *, #17023, .F. ) ;
#61414=DIRECTION ( 'NONE',  ( 1.000000000000000000, 0.000000000000000000, 0.000000000000000000 ) ) ;
#61457=DIRECTION ( 'NONE',  ( 1.000000000000000000, 0.000000000000000000, 0.000000000000000000 ) ) ;
#61496=DIRECTION ( 'NONE',  ( 1.000000000000000000, 0.000000000000000000, 0.000000000000000000 ) ) ;
#61672=LINE ( 'NONE', #55083, #18709 ) ;
#61678=CARTESIAN_POINT ( 'NONE',  ( 60.00000000000000000, 0.000000000000000000, 5.000000000000000000 ) ) ;
#61781=VERTEX_POINT ( 'NONE', #8513 ) ;
#61800=EDGE_LOOP ( 'NONE', ( #64124, #10545 ) ) ;
#61964=EDGE_LOOP ( 'NONE', ( #66467, #1200, #27887, #42161 ) ) ;
#62177=CYLINDRICAL_SURFACE ( 'NONE', #2298, 10.00000000000000000 ) ;
#62339=CIRCLE ( 'NONE', #49984, 89.99999999999998579 ) ;
#62447=ORIENTED_EDGE ( 'NONE', *, *, #7463, .T. ) ;
#62521=ORIENTED_EDGE ( 'NONE', *, *, #14075, .T. ) ;
#62671=AXIS2_PLACEMENT_3D ( 'NONE', #59359, #32638, #54063 ) ;
#62851=DIRECTION ( 'NONE',  ( 0.000000000000000000, 0.000000000000000000, 1.000000000000000000 ) ) ;
#62933=CARTESIAN_POINT ( 'NONE',  ( 0.000000000000000000, 0.000000000000000000, 7.000000000000000000 ) ) ;
#63152=CARTESIAN_POINT ( 'NONE',  ( -34.39004539972345498, 0.000000000000000000, 5.000000000000000000 ) ) ;
#63279=FACE_OUTER_BOUND ( 'NONE', #26855, .T. ) ;
#63335=COLOUR_RGB ( '',0.7921568627450980005, 0.8196078431372548767, 0.9333333333333333481 ) ;
#63523=EDGE_CURVE ( 'NONE', #39998, #23524, #45859, .T. ) ;
#63564=CARTESIAN_POINT ( 'NONE',  ( -24.39004539972345498, 0.000000000000000000, 5.000000000000000000 ) ) ;
#63673=CARTESIAN_POINT ( 'NONE',  ( -89.99999999999998579, 1.102182119232617596E-14, -7.000000000000000000 ) ) ;
#63768=DIRECTION ( 'NONE',  ( 0.000000000000000000, 0.000000000000000000, 1.000000000000000000 ) ) ;
#63868=EDGE_LOOP ( 'NONE', ( #25312, #55846, #27936, #54520 ) ) ;
#63954=FACE_OUTER_BOUND ( 'NONE', #13918, .T. ) ;
#64046=ORIENTED_EDGE ( 'NONE', *, *, #52805, .F. ) ;
#64054=EDGE_CURVE ( 'NONE', #56182, #9547, #68358, .T. ) ;
#64124=ORIENTED_EDGE ( 'NONE', *, *, #40347, .F. ) ;
#64141=EDGE_CURVE ( 'NONE', #56268, #50425, #21199, .T. ) ;
#64145=CARTESIAN_POINT ( 'NONE',  ( 0.000000000000000000, 0.000000000000000000, -10.00000000000000000 ) ) ;
#64168=CYLINDRICAL_SURFACE ( 'NONE', #41564, 10.00000000000000178 ) ;
#64197=FACE_OUTER_BOUND ( 'NONE', #26729, .T. ) ;
#64406=EDGE_CURVE ( 'NONE', #11248, #12451, #14523, .T. ) ;
#64454=DIRECTION ( 'NONE',  ( 1.000000000000000000, 0.000000000000000000, 0.000000000000000000 ) ) ;
#64479=AXIS2_PLACEMENT_3D ( 'NONE', #57531, #42035, #20233 ) ;
#64737=ORIENTED_EDGE ( 'NONE', *, *, #16686, .F. ) ;
#64816=DIRECTION ( 'NONE',  ( -0.000000000000000000, -0.000000000000000000, 1.000000000000000000 ) ) ;
#64868=DIRECTION ( 'NONE',  ( 0.000000000000000000, 0.000000000000000000, 1.000000000000000000 ) ) ;
#64920=DIRECTION ( 'NONE',  ( -0.000000000000000000, -0.000000000000000000, 1.000000000000000000 ) ) ;
#65020=EDGE_CURVE ( 'NONE', #6794, #23524, #30392, .T. ) ;
#65119=CARTESIAN_POINT ( 'NONE',  ( 0.000000000000000000, 0.000000000000000000, -10.00000000000000000 ) ) ;
#65175=VERTEX_POINT ( 'NONE', #26496 ) ;
#65401=EDGE_LOOP ( 'NONE', ( #57904, #47098 ) ) ;
#65487=FACE_OUTER_BOUND ( 'NONE', #31582, .T. ) ;
#65493=DIRECTION ( 'NONE',  ( -0.000000000000000000, -0.000000000000000000, 1.000000000000000000 ) ) ;
#65645=DIRECTION ( 'NONE',  ( 0.000000000000000000, 0.000000000000000000, 1.000000000000000000 ) ) ;
#65776=FACE_OUTER_BOUND ( 'NONE', #61964, .T. ) ;
#65780=FILL_AREA_STYLE_COLOUR ( '', #63335 ) ;
#65782=DIRECTION ( 'NONE',  ( 0.000000000000000000, 0.000000000000000000, -1.000000000000000000 ) ) ;
#66024=DIRECTION ( 'NONE',  ( -0.000000000000000000, -0.000000000000000000, 1.000000000000000000 ) ) ;
#66039=DIRECTION ( 'NONE',  ( 0.000000000000000000, 0.000000000000000000, -1.000000000000000000 ) ) ;
#66133=ORIENTED_EDGE ( 'NONE', *, *, #46300, .F. ) ;
#66355=CARTESIAN_POINT ( 'NONE',  ( 35.39413431650373099, 0.000000000000000000, 5.000000000000000000 ) ) ;
#66467=ORIENTED_EDGE ( 'NONE', *, *, #7047, .T. ) ;
#66482=CARTESIAN_POINT ( 'NONE',  ( 0.000000000000000000, -31.50328976398030534, -5.000000000000000000 ) ) ;
#66502=EDGE_CURVE ( 'NONE', #9869, #45363, #33611, .T. ) ;
#66543=CLOSED_SHELL ( 'NONE', ( #151, #56880, #43562, #8432, #14504, #53655, #53321, #35433, #21837, #49864, #35900, #30612, #34740, #24889, #3254, #66732, #47374, #8359, #56388, #29235, #68693, #51545, #38501, #42473, #6410, #40362, #9353, #24314 ) ) ;
#66732=ADVANCED_FACE ( 'NONE', ( #56979, #29537 ), #40785, .T. ) ;
#66832=AXIS2_PLACEMENT_3D ( 'NONE', #50530, #44558, #8319 ) ;
#66917=CIRCLE ( 'NONE', #29840, 60.00000000000000000 ) ;
#66948=VERTEX_POINT ( 'NONE', #58008 ) ;
#67194=EDGE_CURVE ( 'NONE', #47684, #68905, #16809, .T. ) ;
#67288=DIRECTION ( 'NONE',  ( 0.000000000000000000, 0.000000000000000000, 1.000000000000000000 ) ) ;
#67441=DIRECTION ( 'NONE',  ( 1.000000000000000000, 0.000000000000000000, 0.000000000000000000 ) ) ;
#67617=CIRCLE ( 'NONE', #4684, 75.31295361348104223 ) ;
#67726=LINE ( 'NONE', #57167, #41147 ) ;
#67767=PRODUCT_CONTEXT ( 'NONE', #38134, 'mechanical' ) ;
#67778=CARTESIAN_POINT ( 'NONE',  ( -60.00000000000000000, 7.347880794884118356E-15, 10.00000000000000000 ) ) ;
#67797=CYLINDRICAL_SURFACE ( 'NONE', #30849, 10.00000000000000178 ) ;
#67970=ORIENTED_EDGE ( 'NONE', *, *, #60306, .T. ) ;
#68043=ORIENTED_EDGE ( 'NONE', *, *, #46538, .T. ) ;
#68075=DIRECTION ( 'NONE',  ( -0.000000000000000000, -0.000000000000000000, 1.000000000000000000 ) ) ;
#68148=ORIENTED_EDGE ( 'NONE', *, *, #1694, .F. ) ;
#68190=CARTESIAN_POINT ( 'NONE',  ( 75.31295361348102801, 0.000000000000000000, 2.500000000000030198 ) ) ;
#68335=ORIENTED_EDGE ( 'NONE', *, *, #33142, .F. ) ;
#68356=UNCERTAINTY_MEASURE_WITH_UNIT (LENGTH_MEASURE( 1.000000000000000082E-05 ), #36345, 'distance_accuracy_value', 'NONE');
#68358=CIRCLE ( 'NONE', #14430, 60.00000000000000000 ) ;
#68527=FACE_BOUND ( 'NONE', #45232, .T. ) ;
#68545=ORIENTED_EDGE ( 'NONE', *, *, #11819, .T. ) ;
#68611=EDGE_LOOP ( 'NONE', ( #64046, #2581, #56700, #36436 ) ) ;
#68618=VERTEX_POINT ( 'NONE', #1462 ) ;
#68693=ADVANCED_FACE ( 'NONE', ( #65487 ), #61, .F. ) ;
#68763=CARTESIAN_POINT ( 'NONE',  ( -60.00000000000000000, 0.000000000000000000, -5.000000000000000000 ) ) ;
#68905=VERTEX_POINT ( 'NONE', #63673 ) ;
#69099=FACE_OUTER_BOUND ( 'NONE', #7976, .T. ) ;
#69156=CARTESIAN_POINT ( 'NONE',  ( 10.00000000000000178, 35.26862320190615208, -5.000000000000000000 ) ) ;
#69423=DIRECTION ( 'NONE',  ( 1.000000000000000000, 0.000000000000000000, 0.000000000000000000 ) ) ;
#69449=ORIENTED_EDGE ( 'NONE', *, *, #47864, .T. ) ;
ENDSEC;
END-ISO-10303-21;
